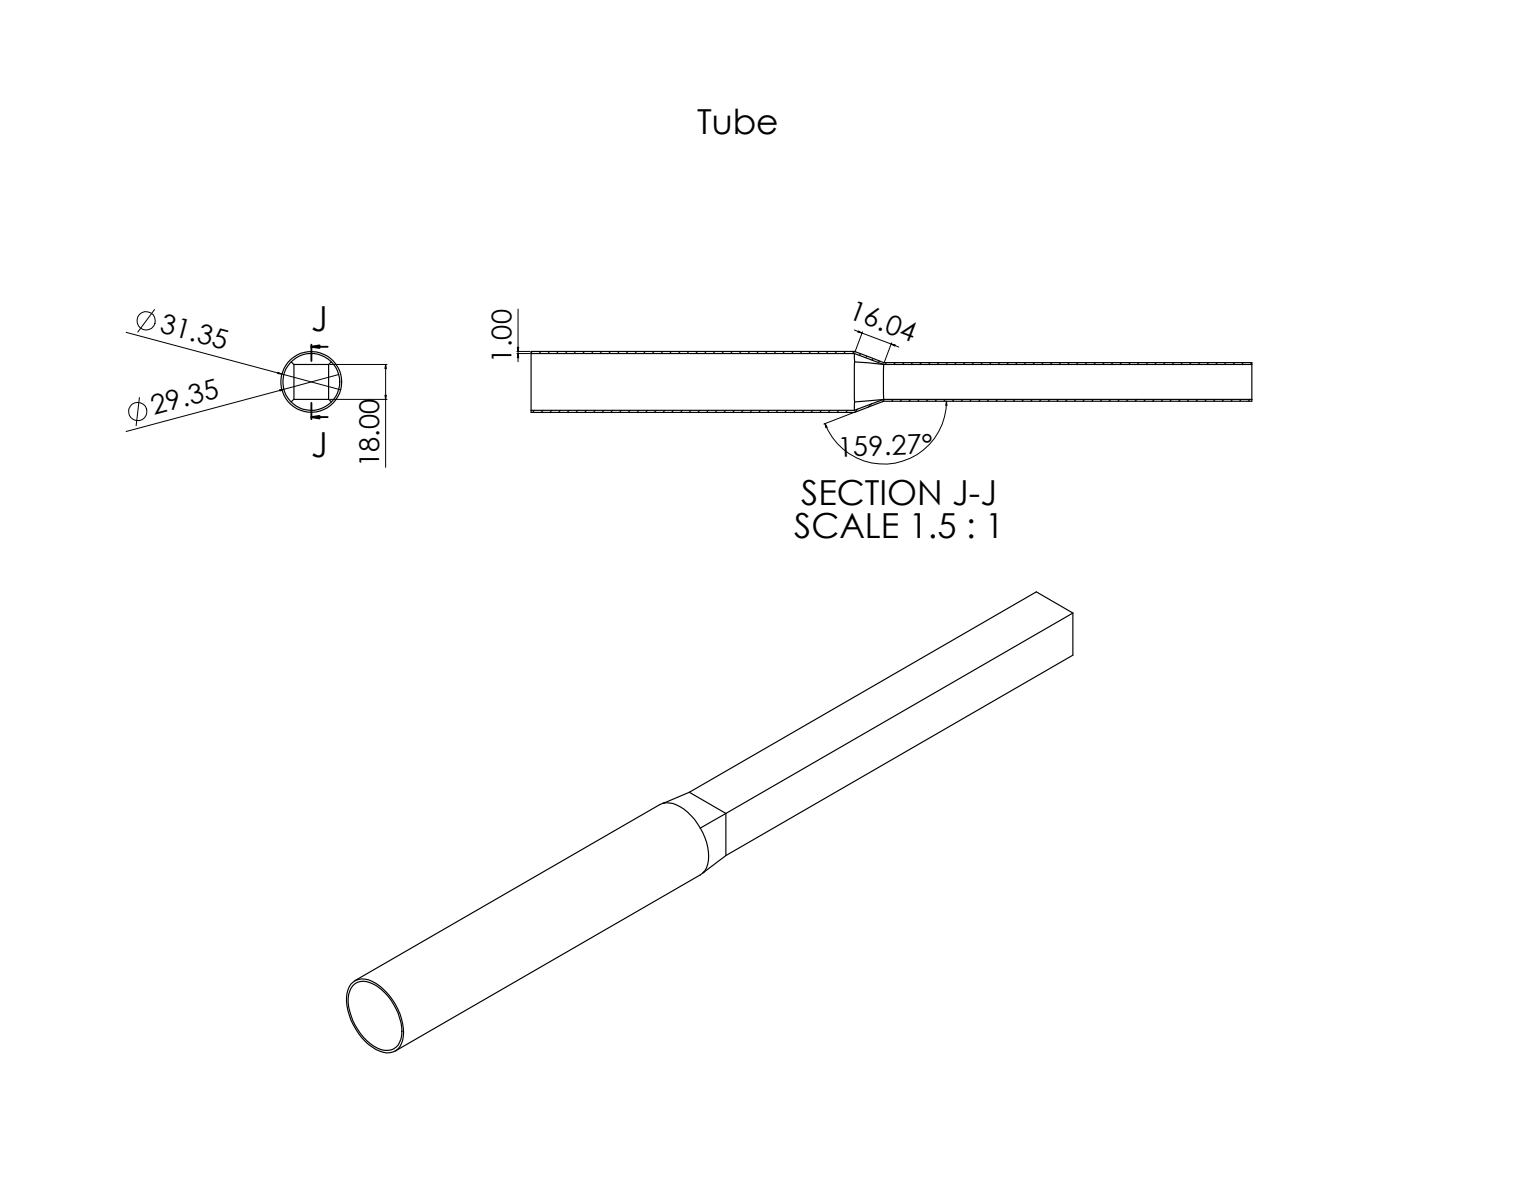
ISO-10303-21;
HEADER;
FILE_DESCRIPTION (('STEP AP214'),
    '1' );
FILE_NAME ('tube.step',
    '2026-10-25T19:19:31',
    ( '' ),
    ( '' ),
    'SwSTEP 2.0',
    'SolidWorks 2025',
    '' );
FILE_SCHEMA (( 'AUTOMOTIVE_DESIGN' ));
ENDSEC;

DATA;
#1=FACE_OUTER_BOUND ( 'NONE', #2199, .T. ) ;
#3=CARTESIAN_POINT ( 'NONE',  ( 6.000509662810415534, -9.000000000000001776, 23.13502399099470708 ) ) ;
#7=CYLINDRICAL_SURFACE ( 'NONE', #5135, 14.67638808697554964 ) ;
#8=ADVANCED_FACE ( 'NONE', ( #6005 ), #1741, .T. ) ;
#10=( NAMED_UNIT ( * ) SI_UNIT ( $, .STERADIAN. ) SOLID_ANGLE_UNIT ( ) );
#14=CARTESIAN_POINT ( 'NONE',  ( 4.154428044945162490, -8.963431230391421423, 23.04275563843252783 ) ) ;
#18=PLANE ( 'NONE',  #4619 ) ;
#25=CARTESIAN_POINT ( 'NONE',  ( 4.399209358691966720, 10.59950146047779995, 28.13666863833444154 ) ) ;
#26=CARTESIAN_POINT ( 'NONE',  ( -0.8333333333332849646, 10.00000000000000000, 23.00000000000000355 ) ) ;
#31=CARTESIAN_POINT ( 'NONE',  ( -9.557272410707511767, 9.557272410707513544, 28.03893107092313031 ) ) ;
#38=CARTESIAN_POINT ( 'NONE',  ( 10.37777353962609972, -10.37777353962564852, 38.05103295300747845 ) ) ;
#39=CARTESIAN_POINT ( 'NONE',  ( 5.954763795926170999, -9.638809746143389035, 25.54536317066256856 ) ) ;
#47=CARTESIAN_POINT ( 'NONE',  ( 9.858401829237470437, -10.19494410001831142, 33.01259202755186095 ) ) ;
#49=ORIENTED_EDGE ( 'NONE', *, *, #1979, .T. ) ;
#50=CARTESIAN_POINT ( 'NONE',  ( 1.902388932222473850, 12.74242197681752486, 33.26151580524048512 ) ) ;
#51=CARTESIAN_POINT ( 'NONE',  ( 11.08488032081242380, 11.08488032081242025, 38.00000000000000000 ) ) ;
#56=ADVANCED_FACE ( 'NONE', ( #3401 ), #273, .T. ) ;
#57=CARTESIAN_POINT ( 'NONE',  ( -10.12138240269938905, -10.27356722921338950, 35.55812462721154787 ) ) ;
#59=STYLED_ITEM('',(#6177),#4119);
#64=CARTESIAN_POINT ( 'NONE',  ( -3.819063922341606521, -14.20304409106748977, 38.16887386538299154 ) ) ;
#66=ORIENTED_EDGE ( 'NONE', *, *, #1371, .T. ) ;
#73=AXIS2_PLACEMENT_3D ( 'NONE', #3304, #3763, #5645 ) ;
#74=CARTESIAN_POINT ( 'NONE',  ( 3.019346778933465369, -14.42236408824967420, 38.33740271606986738 ) ) ;
#87=CARTESIAN_POINT ( 'NONE',  ( -1.016991241531515433, 14.74111653287705792, 38.35393095385146012 ) ) ;
#102=CARTESIAN_POINT ( 'NONE',  ( 0.000000000000000000, 0.000000000000000000, 205.0000000000000568 ) ) ;
#109=CARTESIAN_POINT ( 'NONE',  ( 6.925838250501021420, -10.16165675636470489, 28.06531976343184454 ) ) ;
#115=CARTESIAN_POINT ( 'NONE',  ( -10.37777353962477278, -10.37777353962696303, 38.05103295300743582 ) ) ;
#116=CARTESIAN_POINT ( 'NONE',  ( 10.38144361273100280, -10.38144361273100813, 38.10175261887127363 ) ) ;
#118=PRODUCT_DEFINITION ( 'UNKNOWN', '', #4533, #1451 ) ;
#119=ORIENTED_EDGE ( 'NONE', *, *, #3607, .F. ) ;
#120=CARTESIAN_POINT ( 'NONE',  ( 4.273055220303958457, 9.778265677387498300, 25.59105958838677353 ) ) ;
#121=CARTESIAN_POINT ( 'NONE',  ( 11.73806315776973719, 10.43169748385510687, 38.00000000000000000 ) ) ;
#122=CARTESIAN_POINT ( 'NONE',  ( -13.19705249345109088, -6.492124056757525352, 38.13875458540262997 ) ) ;
#125=CARTESIAN_POINT ( 'NONE',  ( -11.58282027941458381, -3.645499761006322892, 30.69674202529823503 ) ) ;
#129=CARTESIAN_POINT ( 'NONE',  ( 8.309552794738946702, -9.958856949317492990, 22.73823205004162773 ) ) ;
#131=CARTESIAN_POINT ( 'NONE',  ( 0.9493919581231019533, -14.67711297304296281, 38.18288466297301653 ) ) ;
#133=CARTESIAN_POINT ( 'NONE',  ( 6.000548030722291593, 8.999999999999994671, 23.13502304888907446 ) ) ;
#137=CARTESIAN_POINT ( 'NONE',  ( 8.328520801854331523, -12.11088206474084572, 38.20782360758020246 ) ) ;
#146=CARTESIAN_POINT ( 'NONE',  ( 0.8581648076837656847, 9.928243323025451872, 25.63579099555280649 ) ) ;
#147=CARTESIAN_POINT ( 'NONE',  ( 2.164213882025735280, 15.56315586465742484, 38.00000000000000711 ) ) ;
#151=CARTESIAN_POINT ( 'NONE',  ( -13.51119013911330491, -2.923529524533183821, 35.79437308157103814 ) ) ;
#153=CARTESIAN_POINT ( 'NONE',  ( -2.164213882025736613, -15.56315586465742484, 38.00000000000000711 ) ) ;
#156=CARTESIAN_POINT ( 'NONE',  ( 8.964680801521355491, 2.491918585145397991, 23.07363600708416129 ) ) ;
#168=CARTESIAN_POINT ( 'NONE',  ( 1.016991241531512769, -14.74111653287705792, 38.35393095385146012 ) ) ;
#172=FACE_OUTER_BOUND ( 'NONE', #5895, .T. ) ;
#176=B_SPLINE_CURVE_WITH_KNOTS ( 'NONE', 3,
 ( #5640, #360, #5088, #1772, #3271, #6050 ),
 .UNSPECIFIED., .F., .F.,
 ( 4, 2, 4 ),
 ( 2.991083261079382436E-05, 0.007589224902417026838, 0.01514853897222325982 ),
 .UNSPECIFIED. ) ;
#180=CARTESIAN_POINT ( 'NONE',  ( 8.999999999999998224, -9.999999999999998224, 23.00000000000000000 ) ) ;
#181=EDGE_CURVE ( 'NONE', #882, #2297, #5215, .T. ) ;
#186=CARTESIAN_POINT ( 'NONE',  ( 5.819377809724670669, 8.963566137365393871, 22.99383900881164067 ) ) ;
#192=CARTESIAN_POINT ( 'NONE',  ( -9.928243323025453648, 3.951802415609825688E-14, 25.63579099555280294 ) ) ;
#194=CARTESIAN_POINT ( 'NONE',  ( -3.317157231508649495, -9.910574073276151807, 22.73823205004162773 ) ) ;
#195=VECTOR ( 'NONE', #4584, 1000.000000000000000 ) ;
#196=CARTESIAN_POINT ( 'NONE',  ( 13.51119013911330669, 2.923529524533184265, 35.79437308157104525 ) ) ;
#198=LINE ( 'NONE', #2374, #5423 ) ;
#203=CARTESIAN_POINT ( 'NONE',  ( 0.8880320553140116369, -10.89081796499577237, 28.17941898721254645 ) ) ;
#205=DIRECTION ( 'NONE',  ( -0.000000000000000000, -0.000000000000000000, -1.000000000000000000 ) ) ;
#207=CARTESIAN_POINT ( 'NONE',  ( 14.30354638250598498, 3.321916882804190951, 38.17191617598167852 ) ) ;
#219=CARTESIAN_POINT ( 'NONE',  ( 9.999999999999998224, -9.999999999999998224, 23.00000000000000000 ) ) ;
#223=CARTESIAN_POINT ( 'NONE',  ( -9.833810162157899271, -3.423816715609353079, 25.60794618818621160 ) ) ;
#224=EDGE_LOOP ( 'NONE', ( #2924, #3585, #2921, #1569, #6030 ) ) ;
#225=CARTESIAN_POINT ( 'NONE',  ( -8.999999999999998224, 8.999999999999998224, 23.00000000000000000 ) ) ;
#226=CARTESIAN_POINT ( 'NONE',  ( 10.78034266696900012, 2.654236408786700085, 28.16346921039841789 ) ) ;
#231=CARTESIAN_POINT ( 'NONE',  ( -4.003063095775588387, -14.21238549857230993, 38.32638145091770809 ) ) ;
#240=ORIENTED_EDGE ( 'NONE', *, *, #5458, .F. ) ;
#243=CARTESIAN_POINT ( 'NONE',  ( 9.322893336083165394, 9.590870124851308631, 27.95908392747358562 ) ) ;
#244=CARTESIAN_POINT ( 'NONE',  ( 9.916251082295017838, -4.147343260682193389, 22.73823205004162418 ) ) ;
#248=EDGE_CURVE ( 'NONE', #5395, #3300, #425, .T. ) ;
#250=CARTESIAN_POINT ( 'NONE',  ( -10.32656711695238094, -6.095798759547100154, 28.09297316833070113 ) ) ;
#251=VERTEX_POINT ( 'NONE', #3860 ) ;
#254=CARTESIAN_POINT ( 'NONE',  ( 10.46302782743270754, 5.247549479766026259, 28.11481907968152427 ) ) ;
#259=CARTESIAN_POINT ( 'NONE',  ( -5.685785403169735019, -12.74411457810409232, 35.74643938915854591 ) ) ;
#260=ORIENTED_EDGE ( 'NONE', *, *, #822, .T. ) ;
#272=CARTESIAN_POINT ( 'NONE',  ( 7.487361748921665061, 8.967351122863068014, 22.92808036848186504 ) ) ;
#273=B_SPLINE_SURFACE_WITH_KNOTS ( 'NONE', 3, 1, ( 
 ( #5313, #2482, #4370 ),
 ( #121, #3896, #1533 ),
 ( #3311, #5219, #957 ),
 ( #690, #3990, #1683 ),
 ( #2657, #4973, #3555 ),
 ( #774, #4553, #3001 ),
 ( #2602, #5904, #5405 ),
 ( #2062, #1619, #5435 ),
 ( #5474, #4431, #5936 ),
 ( #310, #2189, #4491 ),
 ( #5848, #4517, #1567 ),
 ( #745, #1230, #2626 ),
 ( #4940, #1174, #244 ),
 ( #2573, #1596, #3519 ),
 ( #3468, #3492, #5381 ),
 ( #1204, #1145, #5001 ),
 ( #4464, #1120, #3063 ),
 ( #2116, #219, #4911 ) ),
 .UNSPECIFIED., .F., .F., .F.,
 ( 4, 2, 2, 2, 2, 2, 2, 2, 4 ),
 ( 2, 1, 2 ),
 ( 0.000000000000000000, 0.1250000000000000000, 0.2500000000000000000, 0.3750000000000000000, 0.4999999999999999445, 0.6250000000000000000, 0.7500000000000000000, 0.8750000000000000000, 1.000000000000000000 ),
 ( 0.000000000000000000, 1.000000000000000000, 1.017451196663891722 ),
 .UNSPECIFIED. ) ;
#281=CARTESIAN_POINT ( 'NONE',  ( -9.793760812180220654, 8.539139919159236314, 27.99841606626185353 ) ) ;
#293=VECTOR ( 'NONE', #3601, 1000.000000000000000 ) ;
#294=CARTESIAN_POINT ( 'NONE',  ( 2.830884587392746621, -12.60026679007841466, 33.25110354061416018 ) ) ;
#297=VECTOR ( 'NONE', #4183, 1000.000000000000000 ) ;
#298=ORIENTED_EDGE ( 'NONE', *, *, #2594, .T. ) ;
#303=CARTESIAN_POINT ( 'NONE',  ( 15.67638808697555142, 1.919803849290630886E-15, 205.0000000000000568 ) ) ;
#304=CARTESIAN_POINT ( 'NONE',  ( -9.999999999999998224, 1.666666666666715368, 23.00000000000000000 ) ) ;
#306=ORIENTED_EDGE ( 'NONE', *, *, #668, .F. ) ;
#310=CARTESIAN_POINT ( 'NONE',  ( 15.67638808697555142, -1.082228759108216254, 38.00000000000000711 ) ) ;
#314=CARTESIAN_POINT ( 'NONE',  ( 8.964120815521452457, -3.322922547535530846, 23.06129036953744915 ) ) ;
#315=CARTESIAN_POINT ( 'NONE',  ( -10.78034266696900190, 2.654236408786762702, 28.16346921039841078 ) ) ;
#317=CARTESIAN_POINT ( 'NONE',  ( -10.08321815271042432, 9.378998278013591872, 27.91486726096250948 ) ) ;
#323=EDGE_LOOP ( 'NONE', ( #4367, #5379, #3695, #5284 ) ) ;
#325=CARTESIAN_POINT ( 'NONE',  ( -6.737147714782520502, -13.11522978513662530, 38.26633100282688105 ) ) ;
#330=PLANE ( 'NONE',  #3954 ) ;
#333=CARTESIAN_POINT ( 'NONE',  ( -13.97471987708211216, -7.178663235509280760, 37.99999999999999289 ) ) ;
#336=EDGE_LOOP ( 'NONE', ( #5694, #5269, #1258, #942 ) ) ;
#340=( NAMED_UNIT ( * ) PLANE_ANGLE_UNIT ( ) SI_UNIT ( $, .RADIAN. ) );
#341=CARTESIAN_POINT ( 'NONE',  ( 8.965240787521256749, -1.660914622755447212, 23.08598164463087343 ) ) ;
#342=CARTESIAN_POINT ( 'NONE',  ( -11.98089146579573061, 5.533593864557679431, 33.20390238845318720 ) ) ;
#344=CARTESIAN_POINT ( 'NONE',  ( -8.662324224478984647, 10.23352841777492017, 30.54531597708798074 ) ) ;
#351=CARTESIAN_POINT ( 'NONE',  ( -8.539139919159234537, -9.793760812180220654, 27.99841606626185353 ) ) ;
#353=CARTESIAN_POINT ( 'NONE',  ( 10.37777353962609972, -10.37777353962564852, 38.05103295300747845 ) ) ;
#359=CARTESIAN_POINT ( 'NONE',  ( -9.916251082295017838, 4.147343260682193389, 22.73823205004162418 ) ) ;
#360=CARTESIAN_POINT ( 'NONE',  ( 10.19629538392542933, -10.19629538388540446, 35.54424335298407556 ) ) ;
#363=PLANE ( 'NONE',  #2855 ) ;
#365=CARTESIAN_POINT ( 'NONE',  ( 2.411881101062863575, 14.48475173028204566, 38.17746263717076971 ) ) ;
#369=CARTESIAN_POINT ( 'NONE',  ( 12.81596724893641515, -0.9505942623812210224, 33.26667497053200151 ) ) ;
#370=CARTESIAN_POINT ( 'NONE',  ( -8.963566137365393871, 5.819377809724669781, 22.99383900881164067 ) ) ;
#374=CARTESIAN_POINT ( 'NONE',  ( -2.035738251814317223, 14.63232105816060979, 38.34842656511671066 ) ) ;
#380=CARTESIAN_POINT ( 'NONE',  ( -9.419333092093008730, -9.933255351449998827, 30.50691708577706152 ) ) ;
#384=ORIENTED_EDGE ( 'NONE', *, *, #2250, .F. ) ;
#388=CARTESIAN_POINT ( 'NONE',  ( -9.999999999999998224, 6.666666666666692720, 23.00000000000000000 ) ) ;
#399=CARTESIAN_POINT ( 'NONE',  ( 14.63234267792704557, -2.035630462091353898, 38.34842398122204798 ) ) ;
#402=CARTESIAN_POINT ( 'NONE',  ( -9.908812303639313868, 1.716658579843643118, 25.63028407385522911 ) ) ;
#405=CARTESIAN_POINT ( 'NONE',  ( -8.321944142006520551, 8.970286642449650572, 22.89273687632151066 ) ) ;
#412=CARTESIAN_POINT ( 'NONE',  ( -8.926511697459380557, -11.12726264164139600, 35.63515070857870626 ) ) ;
#420=CARTESIAN_POINT ( 'NONE',  ( -13.47611570251764590, -8.069545871843427420, 37.99999999999998579 ) ) ;
#423=CARTESIAN_POINT ( 'NONE',  ( -9.999999999999998224, -9.999999999999998224, 23.00000000000000000 ) ) ;
#425=LINE ( 'NONE', #3727, #495 ) ;
#427=CARTESIAN_POINT ( 'NONE',  ( 11.85339260696609109, 0.9193131588475963456, 30.72304697887226510 ) ) ;
#430=CARTESIAN_POINT ( 'NONE',  ( -5.685785403169716368, 12.74411457810409587, 35.74643938915853880 ) ) ;
#436=CARTESIAN_POINT ( 'NONE',  ( -10.63625351335941538, -9.632247231687289357, 35.59852902770368388 ) ) ;
#437=CARTESIAN_POINT ( 'NONE',  ( -14.67638808697506114, 0.4806947631990008407, 38.18288438803430296 ) ) ;
#450=ORIENTED_EDGE ( 'NONE', *, *, #856, .T. ) ;
#452=FACE_OUTER_BOUND ( 'NONE', #336, .T. ) ;
#453=CARTESIAN_POINT ( 'NONE',  ( -0.9493919581226956117, 14.67711297304298768, 38.18288466297298811 ) ) ;
#458=CARTESIAN_POINT ( 'NONE',  ( -3.423816715609354411, 9.833810162157899271, 25.60794618818621160 ) ) ;
#464=VERTEX_POINT ( 'NONE', #2022 ) ;
#467=CARTESIAN_POINT ( 'NONE',  ( -8.983694681928700021, -9.994658916190591214, 22.80938439471025703 ) ) ;
#486=CARTESIAN_POINT ( 'NONE',  ( 5.533593864557655451, -11.98089146579573061, 33.20390238845318720 ) ) ;
#487=APPLICATION_CONTEXT ( 'automotive_design' ) ;
#488=EDGE_LOOP ( 'NONE', ( #3553, #1325 ) ) ;
#490=FACE_OUTER_BOUND ( 'NONE', #2075, .T. ) ;
#495=VECTOR ( 'NONE', #5181, 1000.000000000000000 ) ;
#497=CARTESIAN_POINT ( 'NONE',  ( 9.590870124851305079, -9.322893336083168947, 27.95908392747358562 ) ) ;
#498=VECTOR ( 'NONE', #1818, 1000.000000000000000 ) ;
#500=CARTESIAN_POINT ( 'NONE',  ( 4.003063095775587499, 14.21238549857231170, 38.32638145091770809 ) ) ;
#502=CARTESIAN_POINT ( 'NONE',  ( 0.8333333333333816650, 9.999999999999998224, 23.00000000000000000 ) ) ;
#514=CARTESIAN_POINT ( 'NONE',  ( 10.99573437649350538, 9.772747244158498603, 38.14042781937034476 ) ) ;
#515=CARTESIAN_POINT ( 'NONE',  ( 4.709709529607406964, -13.90855959397108954, 38.16103891068024012 ) ) ;
#523=CARTESIAN_POINT ( 'NONE',  ( 9.245260337044127752, -9.269614772507658529, 25.40693856330804934 ) ) ;
#526=CARTESIAN_POINT ( 'NONE',  ( -9.999999999999998224, -9.999999999999998224, 23.00000000000000000 ) ) ;
#532=CARTESIAN_POINT ( 'NONE',  ( 9.933255351449995274, -9.419333092093014059, 30.50691708577705796 ) ) ;
#534=CARTESIAN_POINT ( 'NONE',  ( 6.095889600840177280, 10.32655419438761690, 28.09296952102860701 ) ) ;
#535=CARTESIAN_POINT ( 'NONE',  ( 6.642184745761470666, 9.939337621248920840, 22.73823205004162418 ) ) ;
#539=CARTESIAN_POINT ( 'NONE',  ( -10.38144361273100635, -10.38144361273100458, 38.10175261887127363 ) ) ;
#541=DIRECTION ( 'NONE',  ( -0.000000000000000000, -0.000000000000000000, -1.000000000000000000 ) ) ;
#542=CARTESIAN_POINT ( 'NONE',  ( 9.676903716103607778, -11.04476983075560348, 38.07288907902118069 ) ) ;
#547=CARTESIAN_POINT ( 'NONE',  ( 12.71058384521441198, -7.353037798771444145, 38.12486502407008970 ) ) ;
#548=CARTESIAN_POINT ( 'NONE',  ( 4.954970571217797826, -13.90079966151758306, 38.30990426830500439 ) ) ;
#562=CARTESIAN_POINT ( 'NONE',  ( -0.9833031778629136577, 13.77854189090673742, 35.81030296219172726 ) ) ;
#569=CARTESIAN_POINT ( 'NONE',  ( -11.71459457793454995, -6.400384853991337941, 33.18278774224378225 ) ) ;
#572=CARTESIAN_POINT ( 'NONE',  ( -9.166666666666673180, -9.999999999999998224, 23.00000000000000000 ) ) ;
#576=DIRECTION ( 'NONE',  ( -0.000000000000000000, -0.000000000000000000, -1.000000000000000000 ) ) ;
#586=CARTESIAN_POINT ( 'NONE',  ( 7.077301327650767249, -10.77711034800893231, 30.61076202992614625 ) ) ;
#587=VECTOR ( 'NONE', #3050, 1000.000000000000000 ) ;
#595=CARTESIAN_POINT ( 'NONE',  ( 10.50531938289192624, -7.869812776064898152, 30.57803900350706527 ) ) ;
#599=CARTESIAN_POINT ( 'NONE',  ( 3.531766105781286580, 10.70751178813581461, 28.15279191876807374 ) ) ;
#605=EDGE_CURVE ( 'NONE', #2868, #2500, #2363, .T. ) ;
#606=CARTESIAN_POINT ( 'NONE',  ( -10.59948853791303414, -4.399300199984967463, 28.13666499103235452 ) ) ;
#610=CARTESIAN_POINT ( 'NONE',  ( -8.333333333333348136, -9.999999999999998224, 23.00000000000000000 ) ) ;
#613=CARTESIAN_POINT ( 'NONE',  ( 10.12138240269938905, 10.27356722921338950, 35.55812462721154787 ) ) ;
#615=CIRCLE ( 'NONE', #5164, 15.67638808697555142 ) ;
#619=CARTESIAN_POINT ( 'NONE',  ( 8.999999999999994671, -3.000437278975552235, 23.18288419282212587 ) ) ;
#621=CARTESIAN_POINT ( 'NONE',  ( 5.247549479766027147, -10.46302782743270754, 28.11481907968152427 ) ) ;
#624=ORIENTED_EDGE ( 'NONE', *, *, #3473, .T. ) ;
#628=CARTESIAN_POINT ( 'NONE',  ( -10.19629538388490353, -10.19629538392591428, 35.54424335298404714 ) ) ;
#632=CARTESIAN_POINT ( 'NONE',  ( 0.8880320553140821360, 10.89081796499577059, 28.17941898721253580 ) ) ;
#633=CARTESIAN_POINT ( 'NONE',  ( 7.178663235509286977, 13.97471987708211394, 38.00000000000000000 ) ) ;
#638=CARTESIAN_POINT ( 'NONE',  ( -13.68733454931619953, 1.968046268140568156, 35.80501179064255268 ) ) ;
#640=CARTESIAN_POINT ( 'NONE',  ( 3.317157231508561122, -9.910574073276151807, 22.73823205004162773 ) ) ;
#642=CARTESIAN_POINT ( 'NONE',  ( 12.45812449473958949, 3.759289558891020455, 33.24069098933200905 ) ) ;
#646=EDGE_CURVE ( 'NONE', #1950, #464, #2666, .T. ) ;
#647=CARTESIAN_POINT ( 'NONE',  ( 2.742560498089724241, -11.69030472852370828, 30.70728637550628903 ) ) ;
#654=CARTESIAN_POINT ( 'NONE',  ( 0.000000000000000000, 0.000000000000000000, 38.00000000000000000 ) ) ;
#657=ORIENTED_EDGE ( 'NONE', *, *, #2551, .F. ) ;
#663=CARTESIAN_POINT ( 'NONE',  ( -12.60026679007840933, -2.830884587392748397, 33.25110354061415308 ) ) ;
#664=ORIENTED_EDGE ( 'NONE', *, *, #2969, .F. ) ;
#665=CARTESIAN_POINT ( 'NONE',  ( 1.082228759108211813, -15.67638808697554786, 38.00000000000000711 ) ) ;
#668=EDGE_CURVE ( 'NONE', #5813, #4909, #2649, .T. ) ;
#669=CARTESIAN_POINT ( 'NONE',  ( 12.74240908541723805, 1.902479615894477449, 33.26151609189631841 ) ) ;
#671=CARTESIAN_POINT ( 'NONE',  ( 8.999999999988068211, 9.000000000000005329, 23.06137295785747554 ) ) ;
#675=EDGE_CURVE ( 'NONE', #4909, #1654, #1700, .T. ) ;
#676=CARTESIAN_POINT ( 'NONE',  ( -4.273055220303960233, -9.778265677387510735, 25.59105958838677708 ) ) ;
#684=( GEOMETRIC_REPRESENTATION_CONTEXT ( 3 ) GLOBAL_UNCERTAINTY_ASSIGNED_CONTEXT ( ( #3684 ) ) GLOBAL_UNIT_ASSIGNED_CONTEXT ( ( #1802, #340, #1744 ) ) REPRESENTATION_CONTEXT ( 'NONE', 'WORKASPACE' ) );
#689=CARTESIAN_POINT ( 'NONE',  ( 8.159736356077655017, 11.57174281757876955, 35.66679457777021156 ) ) ;
#690=CARTESIAN_POINT ( 'NONE',  ( 13.47611570251764768, 8.069545871843432749, 37.99999999999999289 ) ) ;
#692=ORIENTED_EDGE ( 'NONE', *, *, #2352, .F. ) ;
#694=CARTESIAN_POINT ( 'NONE',  ( -12.81596724893641337, 1.499651672263871603E-14, 33.26667497053200151 ) ) ;
#696=ORIENTED_EDGE ( 'NONE', *, *, #3568, .F. ) ;
#702=CARTESIAN_POINT ( 'NONE',  ( 9.708537589994000072, 5.113933401365464704, 25.56820946177495557 ) ) ;
#711=CARTESIAN_POINT ( 'NONE',  ( -1.117102909420315718E-14, -13.77854189090673742, 35.81030296219173437 ) ) ;
#714=CARTESIAN_POINT ( 'NONE',  ( 14.58318388806640442, 1.909955344851026027, 38.18050947768620063 ) ) ;
#716=ADVANCED_FACE ( 'NONE', ( #885 ), #3690, .T. ) ;
#717=CARTESIAN_POINT ( 'NONE',  ( -10.00265588554885454, -10.00265588554885454, 33.03935750738951782 ) ) ;
#721=CARTESIAN_POINT ( 'NONE',  ( 7.610208295502498999, 9.462636878983097688, 25.48187184588751464 ) ) ;
#725=CARTESIAN_POINT ( 'NONE',  ( -8.964120776013636771, -3.322926169935023655, 23.06129021161080317 ) ) ;
#728=CARTESIAN_POINT ( 'NONE',  ( 13.50805179034378689, 5.845970755595363499, 38.28811402100272687 ) ) ;
#733=CARTESIAN_POINT ( 'NONE',  ( -4.807771419025854698, -13.07374771013670411, 35.76776546669864132 ) ) ;
#735=CARTESIAN_POINT ( 'NONE',  ( -8.999999999999994671, 3.000437278975516708, 23.18288419282211521 ) ) ;
#744=CARTESIAN_POINT ( 'NONE',  ( 9.632247231687292910, 10.63625351335941716, 35.59852902770369809 ) ) ;
#745=CARTESIAN_POINT ( 'NONE',  ( 15.12434353048566571, -4.260267006495016773, 38.00000000000000711 ) ) ;
#746=CARTESIAN_POINT ( 'NONE',  ( -15.67638808697555142, -2.609965535188016420E-15, 38.00000000000000711 ) ) ;
#750=CARTESIAN_POINT ( 'NONE',  ( -10.67320828294309898, 8.785766938566926143, 33.09220912812762094 ) ) ;
#752=CARTESIAN_POINT ( 'NONE',  ( -10.27356722921338950, 10.12138240269938905, 35.55812462721154787 ) ) ;
#754=CARTESIAN_POINT ( 'NONE',  ( 10.23352841777492017, 8.662324224478986423, 30.54531597708798074 ) ) ;
#758=B_SPLINE_CURVE_WITH_KNOTS ( 'NONE', 3,
 ( #38, #2893, #943, #4797, #547, #2366, #1364, #5699, #2425, #1916, #4261, #3269, #2864, #4768 ),
 .UNSPECIFIED., .F., .F.,
 ( 4, 2, 2, 2, 2, 2, 4 ),
 ( 2.453269466693398698E-18, 0.002860246893306488992, 0.004290370339959730453, 0.005720493786612971913, 0.008580740679919452232, 0.01001086412657269456, 0.01144098757322593515 ),
 .UNSPECIFIED. ) ;
#760=CARTESIAN_POINT ( 'NONE',  ( -3.759380242563084451, -12.45811160333930800, 33.24069127598783524 ) ) ;
#761=ORIENTED_EDGE ( 'NONE', *, *, #4032, .F. ) ;
#766=VECTOR ( 'NONE', #3692, 1000.000000000000000 ) ;
#768=PRODUCT_CONTEXT ( 'NONE', #487, 'mechanical' ) ;
#770=CARTESIAN_POINT ( 'NONE',  ( -9.969668718019493170, -9.144590365090015993, 22.73823205004162418 ) ) ;
#774=CARTESIAN_POINT ( 'NONE',  ( 14.79903580929011753, 5.273949241992679227, 38.00000000000000711 ) ) ;
#779=ADVANCED_FACE ( 'NONE', ( #5517 ), #330, .T. ) ;
#783=CARTESIAN_POINT ( 'NONE',  ( -10.99573437649350183, 9.772747244158500379, 38.14042781937034476 ) ) ;
#785=CARTESIAN_POINT ( 'NONE',  ( -9.772747244158496827, 10.99573437649350538, 38.14042781937034476 ) ) ;
#795=CARTESIAN_POINT ( 'NONE',  ( -7.228600378928581982, -11.39263409468387422, 33.15620577507543487 ) ) ;
#801=CARTESIAN_POINT ( 'NONE',  ( 0.000000000000000000, 0.000000000000000000, 38.00000000000000000 ) ) ;
#805=CARTESIAN_POINT ( 'NONE',  ( -9.999999999999998224, 3.333333333333377890, 23.00000000000000000 ) ) ;
#814=CARTESIAN_POINT ( 'NONE',  ( 13.77854189090674097, -0.9833031778629309771, 35.81030296219172726 ) ) ;
#815=CARTESIAN_POINT ( 'NONE',  ( -11.03292118881348394, 8.007183658747754507, 33.12420745160153501 ) ) ;
#817=CARTESIAN_POINT ( 'NONE',  ( -6.248091806769195955, 11.02058084744346189, 30.63788045528724524 ) ) ;
#820=CARTESIAN_POINT ( 'NONE',  ( 8.999999999999994671, 6.000509662810391553, 23.13502399099459339 ) ) ;
#822=EDGE_CURVE ( 'NONE', #5813, #2500, #2325, .T. ) ;
#826=CARTESIAN_POINT ( 'NONE',  ( -7.487361748921665061, -8.967351122863068014, 22.92808036848186859 ) ) ;
#834=CARTESIAN_POINT ( 'NONE',  ( -9.999999999999998224, 5.833333333333365012, 23.00000000000000000 ) ) ;
#839=CARTESIAN_POINT ( 'NONE',  ( -6.488003555186317328, 13.19914683770227093, 38.13881399654477633 ) ) ;
#840=CARTESIAN_POINT ( 'NONE',  ( 10.85317354580219629, -1.776706711792237492, 28.17414650202875137 ) ) ;
#841=CARTESIAN_POINT ( 'NONE',  ( -8.963498645742985715, 4.986905650496099796, 23.01829711214647745 ) ) ;
#843=CARTESIAN_POINT ( 'NONE',  ( -5.390571672161838634, 11.22195964661421819, 30.65936073406735574 ) ) ;
#846=CARTESIAN_POINT ( 'NONE',  ( -14.65251043020005461, 0.9663357036150521662, 38.18273246053422554 ) ) ;
#856=EDGE_CURVE ( 'NONE', #1594, #1863, #4862, .T. ) ;
#857=CARTESIAN_POINT ( 'NONE',  ( -15.12434353048566216, -4.260267006495012332, 37.99999999999999289 ) ) ;
#863=CARTESIAN_POINT ( 'NONE',  ( -11.08488032081242558, -11.08488032081241847, 38.00000000000000000 ) ) ;
#864=CARTESIAN_POINT ( 'NONE',  ( 1.937269431830858979, 14.55597330376932774, 38.18000980160653768 ) ) ;
#865=CARTESIAN_POINT ( 'NONE',  ( 13.07374771013670589, -4.807771419025858251, 35.76776546669863421 ) ) ;
#866=VECTOR ( 'NONE', #2323, 1000.000000000000000 ) ;
#867=CARTESIAN_POINT ( 'NONE',  ( -12.24723121994939135, 4.666652649023722788, 33.22501677959694177 ) ) ;
#871=CARTESIAN_POINT ( 'NONE',  ( -7.869812776064877724, 10.50531938289192624, 30.57803900350706172 ) ) ;
#879=CARTESIAN_POINT ( 'NONE',  ( -9.322893336083163618, -9.590870124851308631, 27.95908392747358917 ) ) ;
#882=VERTEX_POINT ( 'NONE', #2422 ) ;
#885=FACE_OUTER_BOUND ( 'NONE', #1773, .T. ) ;
#888=CARTESIAN_POINT ( 'NONE',  ( -12.35760627049922000, -9.696021465980068754, 37.99999999999998579 ) ) ;
#891=VECTOR ( 'NONE', #1166, 1000.000000000000000 ) ;
#895=EDGE_CURVE ( 'NONE', #2972, #5932, #3846, .T. ) ;
#900=CARTESIAN_POINT ( 'NONE',  ( 9.778265677387498300, -4.273055220303958457, 25.59105958838677353 ) ) ;
#901=CIRCLE ( 'NONE', #1670, 15.67638808697555142 ) ;
#903=ADVANCED_FACE ( 'NONE', ( #2395 ), #7, .F. ) ;
#904=CARTESIAN_POINT ( 'NONE',  ( -8.432782529159778662, 9.370308598635419983, 25.44727941985334496 ) ) ;
#908=CARTESIAN_POINT ( 'NONE',  ( -14.55721289103182237, 1.928061058260225558, 38.18004976450266952 ) ) ;
#909=CARTESIAN_POINT ( 'NONE',  ( -9.086997423426605991, -11.58116666691846852, 38.17633527770230017 ) ) ;
#910=EDGE_LOOP ( 'NONE', ( #49, #1213, #66, #5315 ) ) ;
#920=DIRECTION ( 'NONE',  ( -0.000000000000000000, -0.000000000000000000, -1.000000000000000000 ) ) ;
#925=CARTESIAN_POINT ( 'NONE',  ( 11.22195964661421641, -5.390571672161878602, 30.65936073406735218 ) ) ;
#928=CARTESIAN_POINT ( 'NONE',  ( -8.328520801854338629, 12.11088206474084750, 38.20782360758020957 ) ) ;
#929=CARTESIAN_POINT ( 'NONE',  ( -11.08488032081242025, 11.08488032081242203, 38.00000000000000000 ) ) ;
#936=VERTEX_POINT ( 'NONE', #3385 ) ;
#942=ORIENTED_EDGE ( 'NONE', *, *, #895, .F. ) ;
#943=CARTESIAN_POINT ( 'NONE',  ( 11.66987820548568600, -8.950926204225938321, 38.09167945787535103 ) ) ;
#944=CARTESIAN_POINT ( 'NONE',  ( 8.432782529159780438, -9.370308598635425312, 25.44727941985334851 ) ) ;
#955=ORIENTED_EDGE ( 'NONE', *, *, #646, .F. ) ;
#956=CARTESIAN_POINT ( 'NONE',  ( 8.830123324796599503E-15, 13.77854189090673742, 35.81030296219172726 ) ) ;
#957=CARTESIAN_POINT ( 'NONE',  ( 9.958856949317492990, 8.309552794738946702, 22.73823205004162418 ) ) ;
#966=CARTESIAN_POINT ( 'NONE',  ( -10.23352841777491840, -8.662324224478982870, 30.54531597708798074 ) ) ;
#973=CARTESIAN_POINT ( 'NONE',  ( 5.161660887237665918, -13.74708875321000789, 38.15586426248330554 ) ) ;
#978=DIRECTION ( 'NONE',  ( 1.000000000000000000, 0.000000000000000000, 0.000000000000000000 ) ) ;
#983=CARTESIAN_POINT ( 'NONE',  ( 3.759289558891017347, -12.45812449473959127, 33.24069098933200195 ) ) ;
#984=ORIENTED_EDGE ( 'NONE', *, *, #4331, .T. ) ;
#994=CARTESIAN_POINT ( 'NONE',  ( 4.666652649023724564, 12.24723121994938779, 33.22501677959694177 ) ) ;
#996=CARTESIAN_POINT ( 'NONE',  ( -3.317157231508560677, 9.910574073276151807, 22.73823205004162418 ) ) ;
#1001=AXIS2_PLACEMENT_3D ( 'NONE', #5430, #3956, #3984 ) ;
#1002=CARTESIAN_POINT ( 'NONE',  ( -9.618700053625529378, -10.13908112636437053, 30.46372964425718521 ) ) ;
#1003=CARTESIAN_POINT ( 'NONE',  ( -6.666666666666693608, -9.999999999999998224, 23.00000000000000000 ) ) ;
#1008=CARTESIAN_POINT ( 'NONE',  ( -7.765009959109524296, -12.46305503907367829, 38.11687012676383546 ) ) ;
#1014=FACE_BOUND ( 'NONE', #3004, .T. ) ;
#1016=CARTESIAN_POINT ( 'NONE',  ( 7.393143600131246274, -12.01612071878465571, 35.69844150329611665 ) ) ;
#1020=DIRECTION ( 'NONE',  ( 0.000000000000000000, 1.000000000000000000, 0.000000000000000000 ) ) ;
#1025=DIRECTION ( 'NONE',  ( 0.000000000000000000, -1.000000000000000000, 0.000000000000000000 ) ) ;
#1026=ORIENTED_EDGE ( 'NONE', *, *, #4032, .T. ) ;
#1027=CARTESIAN_POINT ( 'NONE',  ( 3.080172029080881894E-14, 10.89081796499577237, 28.17941898721253580 ) ) ;
#1028=CARTESIAN_POINT ( 'NONE',  ( -1.657983872361815658, 9.902916272933978803, 22.73823205004162418 ) ) ;
#1032=CARTESIAN_POINT ( 'NONE',  ( -12.01612071878465393, -7.393143600131249826, 35.69844150329610954 ) ) ;
#1033=CARTESIAN_POINT ( 'NONE',  ( -5.809855716632679190, -9.930636381741159369, 22.73823205004162773 ) ) ;
#1034=CARTESIAN_POINT ( 'NONE',  ( -9.306281718482047438, 9.306281718482050991, 25.54332486258997292 ) ) ;
#1035=CARTESIAN_POINT ( 'NONE',  ( -4.735139425639592226, -13.92517021172167624, 38.16137691020122702 ) ) ;
#1037=CARTESIAN_POINT ( 'NONE',  ( -9.999999999999998224, -9.999999999999998224, -167.0000000000000284 ) ) ;
#1040=ADVANCED_FACE ( 'NONE', ( #2741 ), #363, .F. ) ;
#1044=CARTESIAN_POINT ( 'NONE',  ( 5.845970755595360835, -13.50805179034379400, 38.28811402100272687 ) ) ;
#1051=EDGE_CURVE ( 'NONE', #1654, #5395, #2655, .T. ) ;
#1053=CARTESIAN_POINT ( 'NONE',  ( 9.977717576970368540, -7.732441893382042686, 28.03187055541259909 ) ) ;
#1055=ORIENTED_EDGE ( 'NONE', *, *, #1408, .F. ) ;
#1056=CARTESIAN_POINT ( 'NONE',  ( 1.968046268140572819, 13.68733454931619775, 35.80501179064255268 ) ) ;
#1057=CARTESIAN_POINT ( 'NONE',  ( -1.082228759108214478, 15.67638808697554786, 38.00000000000000711 ) ) ;
#1063=CARTESIAN_POINT ( 'NONE',  ( -13.77854189090673742, -0.9833031778629152120, 35.81030296219172726 ) ) ;
#1067=CARTESIAN_POINT ( 'NONE',  ( 9.166666666666657193, -9.999999999999998224, 23.00000000000000000 ) ) ;
#1070=CARTESIAN_POINT ( 'NONE',  ( 8.999999999999998224, 8.999999999999998224, 23.00000000000000000 ) ) ;
#1071=DIRECTION ( 'NONE',  ( 0.000000000000000000, 0.000000000000000000, -1.000000000000000000 ) ) ;
#1079=CARTESIAN_POINT ( 'NONE',  ( 5.819383256046889663, -8.963566061094551785, 22.99383858586043772 ) ) ;
#1084=CARTESIAN_POINT ( 'NONE',  ( 10.54244016040620835, -10.54244016040621190, 30.50000000000000000 ) ) ;
#1087=PLANE ( 'NONE',  #2380 ) ;
#1092=CARTESIAN_POINT ( 'NONE',  ( 5.113933401365548193, 9.708537589994000072, 25.56820946177495557 ) ) ;
#1099=CARTESIAN_POINT ( 'NONE',  ( -13.33506331686137614, -3.878911688431557536, 35.78373290693654951 ) ) ;
#1103=CARTESIAN_POINT ( 'NONE',  ( 9.696021465980065202, -12.35760627049922356, 37.99999999999999289 ) ) ;
#1105=CARTESIAN_POINT ( 'NONE',  ( 14.42236408824967242, 3.019346778933472031, 38.33740271606986738 ) ) ;
#1108=ORIENTED_EDGE ( 'NONE', *, *, #3013, .T. ) ;
#1111=CARTESIAN_POINT ( 'NONE',  ( 1.716690548177164821, -9.908812100099977371, 25.63028262842344773 ) ) ;
#1114=CARTESIAN_POINT ( 'NONE',  ( 10.72018218391672661, 10.03536489533503762, 38.06196296973745774 ) ) ;
#1116=CARTESIAN_POINT ( 'NONE',  ( 9.999999999999998224, 9.999999999999998224, -167.0000000000000284 ) ) ;
#1119=CARTESIAN_POINT ( 'NONE',  ( 6.925743867604852610, 10.16167434176051643, 28.06532504456334109 ) ) ;
#1120=CARTESIAN_POINT ( 'NONE',  ( 9.999999999999998224, -9.166666666666673180, 23.00000000000000000 ) ) ;
#1126=CARTESIAN_POINT ( 'NONE',  ( -9.708537589994000072, -5.113933401365464704, 25.56820946177495912 ) ) ;
#1127=ORIENTED_EDGE ( 'NONE', *, *, #3568, .T. ) ;
#1128=CARTESIAN_POINT ( 'NONE',  ( -9.696021465980074083, -12.35760627049922178, 38.00000000000000000 ) ) ;
#1130=CARTESIAN_POINT ( 'NONE',  ( 13.90079966151757951, 4.954970571217797826, 38.30990426830500439 ) ) ;
#1134=CARTESIAN_POINT ( 'NONE',  ( -2.763109891354090380E-14, -11.85339260696609465, 30.72304697887227221 ) ) ;
#1136=DIRECTION ( 'NONE',  ( 0.000000000000000000, 0.000000000000000000, -1.000000000000000000 ) ) ;
#1138=CARTESIAN_POINT ( 'NONE',  ( -8.999999999999998224, 8.999999999999998224, -167.0000000000000284 ) ) ;
#1144=CARTESIAN_POINT ( 'NONE',  ( 10.13908112636436343, 9.618700053625531154, 30.46372964425718521 ) ) ;
#1145=CARTESIAN_POINT ( 'NONE',  ( 9.999999999999998224, -8.333333333333348136, 23.00000000000000000 ) ) ;
#1147=CARTESIAN_POINT ( 'NONE',  ( -11.42333844578496915, -4.533051537554476873, 30.68084101284746623 ) ) ;
#1148=ORIENTED_EDGE ( 'NONE', *, *, #605, .F. ) ;
#1154=CARTESIAN_POINT ( 'NONE',  ( 10.67327843797381171, 8.785602912694963962, 33.09221060678261495 ) ) ;
#1157=VERTEX_POINT ( 'NONE', #3209 ) ;
#1159=DIRECTION ( 'NONE',  ( 1.000000000000000000, 0.000000000000000000, 0.000000000000000000 ) ) ;
#1160=CARTESIAN_POINT ( 'NONE',  ( -4.721144251037624463E-14, -8.965668681055127820, 23.09216300389307364 ) ) ;
#1162=EDGE_CURVE ( 'NONE', #3749, #1654, #5740, .T. ) ;
#1166=DIRECTION ( 'NONE',  ( -1.000000000000000000, 0.000000000000000000, 0.000000000000000000 ) ) ;
#1171=ORIENTED_EDGE ( 'NONE', *, *, #3645, .F. ) ;
#1173=CARTESIAN_POINT ( 'NONE',  ( 9.086997423426605991, 11.58116666691846852, 38.17633527770230017 ) ) ;
#1174=CARTESIAN_POINT ( 'NONE',  ( 9.999999999999998224, -4.166666666666706931, 23.00000000000000000 ) ) ;
#1177=CARTESIAN_POINT ( 'NONE',  ( -10.70751606408958700, -3.531709963121627105, 28.15279306126447523 ) ) ;
#1181=AXIS2_PLACEMENT_3D ( 'NONE', #102, #4254, #5793 ) ;
#1182=CARTESIAN_POINT ( 'NONE',  ( 8.963566061094550008, 5.819383256046893216, 22.99383858586042351 ) ) ;
#1186=CARTESIAN_POINT ( 'NONE',  ( -9.000000000000005329, 8.999999999988014920, 23.06137295785748265 ) ) ;
#1189=LINE ( 'NONE', #3046, #1580 ) ;
#1191=CARTESIAN_POINT ( 'NONE',  ( -0.9833031778629336417, -13.77854189090673742, 35.81030296219173437 ) ) ;
#1203=CARTESIAN_POINT ( 'NONE',  ( 8.539139919159236314, 9.793760812180218878, 27.99841606626185353 ) ) ;
#1204=CARTESIAN_POINT ( 'NONE',  ( 12.35760627049921823, -9.696021465980074083, 38.00000000000000000 ) ) ;
#1205=PLANE ( 'NONE',  #3442 ) ;
#1208=CARTESIAN_POINT ( 'NONE',  ( -11.58281169573755953, 3.645573174172184405, 30.69674159737795449 ) ) ;
#1212=CARTESIAN_POINT ( 'NONE',  ( 9.793778397576030414, 8.539045536263008884, 27.99842134739334654 ) ) ;
#1213=ORIENTED_EDGE ( 'NONE', *, *, #2517, .T. ) ;
#1214=CARTESIAN_POINT ( 'NONE',  ( -6.666666666666638541, 9.999999999999998224, 23.00000000000000000 ) ) ;
#1215=LINE ( 'NONE', #5487, #3074 ) ;
#1216=CARTESIAN_POINT ( 'NONE',  ( -1.968046268140571486, -13.68733454931619953, 35.80501179064255268 ) ) ;
#1221=ADVANCED_FACE ( 'NONE', ( #490 ), #3821, .T. ) ;
#1225=CARTESIAN_POINT ( 'NONE',  ( -9.999999999999998224, -1.666666666666617225, 23.00000000000000000 ) ) ;
#1230=CARTESIAN_POINT ( 'NONE',  ( 9.999999999999998224, -3.333333333333376558, 23.00000000000000000 ) ) ;
#1231=DIRECTION ( 'NONE',  ( 0.000000000000000000, -1.000000000000000000, 0.000000000000000000 ) ) ;
#1233=CARTESIAN_POINT ( 'NONE',  ( -13.33504572891042272, 3.879012780925821247, 35.78373437249953781 ) ) ;
#1236=DIRECTION ( 'NONE',  ( 0.000000000000000000, 0.000000000000000000, -1.000000000000000000 ) ) ;
#1240=CARTESIAN_POINT ( 'NONE',  ( -8.159736356077658570, -11.57174281757876955, 35.66679457777021156 ) ) ;
#1242=CARTESIAN_POINT ( 'NONE',  ( -8.999999999988011368, -9.000000000000007105, 23.06137295785747909 ) ) ;
#1245=( GEOMETRIC_REPRESENTATION_CONTEXT ( 3 ) GLOBAL_UNCERTAINTY_ASSIGNED_CONTEXT ( ( #4246 ) ) GLOBAL_UNIT_ASSIGNED_CONTEXT ( ( #1819, #3753, #10 ) ) REPRESENTATION_CONTEXT ( 'NONE', 'WORKASPACE' ) );
#1249=CARTESIAN_POINT ( 'NONE',  ( -9.999999999999998224, -5.833333333333296622, 23.00000000000000000 ) ) ;
#1253=DIRECTION ( 'NONE',  ( 0.000000000000000000, 1.000000000000000000, 0.000000000000000000 ) ) ;
#1258=ORIENTED_EDGE ( 'NONE', *, *, #4180, .F. ) ;
#1259=CARTESIAN_POINT ( 'NONE',  ( 12.41448144607148052, -6.563799387313611788, 35.72511331161844339 ) ) ;
#1261=CARTESIAN_POINT ( 'NONE',  ( -9.778265677387498300, 4.273055220303942470, 25.59105958838676997 ) ) ;
#1270=CARTESIAN_POINT ( 'NONE',  ( -9.157688896001754841, -8.975362584346067152, 22.85246612729343596 ) ) ;
#1284=CIRCLE ( 'NONE', #1976, 15.67638808697555142 ) ;
#1286=CARTESIAN_POINT ( 'NONE',  ( 10.89081796499577059, -3.519470773090535588E-14, 28.17941898721253580 ) ) ;
#1287=CARTESIAN_POINT ( 'NONE',  ( -8.964120815521452457, 3.322922547535531734, 23.06129036953744915 ) ) ;
#1289=CARTESIAN_POINT ( 'NONE',  ( -4.154428044945160714, 8.963431230391419646, 23.04275563843252783 ) ) ;
#1294=DIRECTION ( 'NONE',  ( 1.000000000000000000, -0.000000000000000000, 0.000000000000000000 ) ) ;
#1298=B_SPLINE_SURFACE_WITH_KNOTS ( 'NONE', 3, 3, ( 
 ( #5480, #752, #5039, #4056, #317, #2160, #5975 ),
 ( #785, #4498, #4563, #6000, #5536, #5446, #2098 ),
 ( #3528, #2752, #5590, #344, #1873, #904, #405 ),
 ( #928, #2345, #3245, #871, #1346, #1378, #2784 ),
 ( #3676, #4651, #3649, #4680, #3283, #3216, #3768 ),
 ( #5683, #6085, #5070, #817, #1836, #2693, #6062 ),
 ( #2281, #430, #3702, #843, #2309, #4591, #4199 ),
 ( #4235, #2219, #5187, #4110, #6032, #2810, #1289 ),
 ( #1782, #3251, #6115, #4706, #1806, #458, #5565 ),
 ( #1752, #3188, #2719, #5097, #4148, #4617, #2251 ),
 ( #374, #1315, #5123, #4173, #5156, #1968, #4369 ),
 ( #87, #562, #4810, #2441, #3831, #2936, #5810 ),
 ( #1932, #956, #4398, #2973, #1027, #5748, #4747 ),
 ( #5312, #4335, #1410, #5348, #632, #146, #5285 ),
 ( #1532, #1056, #50, #1474, #2906, #1902, #4848 ),
 ( #3372, #2027, #3926, #3310, #3866, #5218, #2842 ),
 ( #500, #4301, #2382, #5783, #599, #1504, #5253 ),
 ( #4273, #2479, #994, #2510, #25, #120, #3797 ),
 ( #3895, #5711, #3400, #2000, #3434, #1092, #4884 ),
 ( #1438, #3340, #2878, #4781, #534, #2412, #186 ),
 ( #2152, #4938, #4490, #5473, #1119, #1682, #2115 ),
 ( #5878, #689, #4516, #4430, #2061, #721, #272 ),
 ( #1173, #3062, #3119, #1595, #1203, #3092, #3491 ),
 ( #5000, #744, #3582, #4045, #243, #2625, #5966 ),
 ( #5404, #5499, #1618, #1144, #4910, #2656, #3467 ) ),
 .UNSPECIFIED., .F., .F., .F.,
 ( 4, 3, 3, 3, 3, 3, 3, 3, 4 ),
 ( 4, 3, 4 ),
 ( 0.000000000000000000, 0.1250000000000000000, 0.2500000000000000000, 0.3750000000000000000, 0.5000000000000000000, 0.6250000000000000000, 0.7500000000000000000, 0.8750000000000000000, 1.000000000000000000 ),
 ( 0.000000000000000000, 0.5087255983319458608, 1.017451196663891722 ),
 .UNSPECIFIED. ) ;
#1304=CARTESIAN_POINT ( 'NONE',  ( -9.999999999999998224, 9.999999999999998224, 23.00000000000000000 ) ) ;
#1306=CARTESIAN_POINT ( 'NONE',  ( -9.999999999999998224, 9.999999999999998224, 23.00000000000000000 ) ) ;
#1311=CARTESIAN_POINT ( 'NONE',  ( -10.37777353962637505, 10.37777353962536608, 38.05103295300745003 ) ) ;
#1312=CARTESIAN_POINT ( 'NONE',  ( 9.928243323025453648, -2.905319074912632839E-14, 25.63579099555277807 ) ) ;
#1313=CARTESIAN_POINT ( 'NONE',  ( -10.77715421822219177, 7.077172123266720405, 30.61076540981939687 ) ) ;
#1315=CARTESIAN_POINT ( 'NONE',  ( -1.968147360634808329, 13.68731696136523546, 35.80501325620552677 ) ) ;
#1324=CARTESIAN_POINT ( 'NONE',  ( -5.247549479766072444, -10.46302782743270932, 28.11481907968152427 ) ) ;
#1325=ORIENTED_EDGE ( 'NONE', *, *, #646, .T. ) ;
#1326=CARTESIAN_POINT ( 'NONE',  ( -9.999999999999998224, -9.999999999999998224, 23.00000000000000000 ) ) ;
#1328=CARTESIAN_POINT ( 'NONE',  ( 14.67638808697554964, 1.797339169375895343E-15, 205.0000000000000568 ) ) ;
#1332=CARTESIAN_POINT ( 'NONE',  ( -9.902916272933978803, 1.657983872361913358, 22.73823205004162418 ) ) ;
#1342=CARTESIAN_POINT ( 'NONE',  ( 10.78034266696900367, -2.654236408786761814, 28.16346921039841433 ) ) ;
#1346=CARTESIAN_POINT ( 'NONE',  ( -7.732441893382013376, 9.977717576970368540, 28.03187055541259198 ) ) ;
#1350=CARTESIAN_POINT ( 'NONE',  ( 8.999999999999992895, 3.000397777471232708, 23.18288458324510515 ) ) ;
#1352=CARTESIAN_POINT ( 'NONE',  ( 15.67638808697555142, 1.919803849290630886E-15, 205.0000000000000568 ) ) ;
#1355=CARTESIAN_POINT ( 'NONE',  ( 11.08488032081242380, 11.08488032081242025, 38.00000000000000000 ) ) ;
#1364=CARTESIAN_POINT ( 'NONE',  ( 13.37091851167925149, -6.070355506015043368, 38.14417062278695880 ) ) ;
#1371=EDGE_CURVE ( 'NONE', #3081, #1401, #4508, .T. ) ;
#1375=CARTESIAN_POINT ( 'NONE',  ( 13.33504572891042095, -3.879012780925821691, 35.78373437249953781 ) ) ;
#1378=CARTESIAN_POINT ( 'NONE',  ( -7.610208295502463471, 9.462636878983097688, 25.48187184588751464 ) ) ;
#1383=CARTESIAN_POINT ( 'NONE',  ( -9.166555234036119160, -10.04707028972859106, 25.36260747786040071 ) ) ;
#1388=CARTESIAN_POINT ( 'NONE',  ( 9.858401829237468661, 10.19494410001831675, 33.01259202755186095 ) ) ;
#1396=DIRECTION ( 'NONE',  ( 0.000000000000000000, 0.000000000000000000, 1.000000000000000000 ) ) ;
#1398=EDGE_CURVE ( 'NONE', #5460, #882, #4987, .T. ) ;
#1401=VERTEX_POINT ( 'NONE', #1138 ) ;
#1407=CARTESIAN_POINT ( 'NONE',  ( 10.77715421822219355, -7.077172123266713299, 30.61076540981938976 ) ) ;
#1408=EDGE_CURVE ( 'NONE', #1157, #2972, #2564, .T. ) ;
#1410=CARTESIAN_POINT ( 'NONE',  ( 0.9505942623812212444, 12.81596724893641337, 33.26667497053200151 ) ) ;
#1416=CARTESIAN_POINT ( 'NONE',  ( -9.370308598635419983, -8.432782529159780438, 25.44727941985334496 ) ) ;
#1417=CARTESIAN_POINT ( 'NONE',  ( 11.08488032081241847, -11.08488032081242380, 38.00000000000000000 ) ) ;
#1419=CARTESIAN_POINT ( 'NONE',  ( 9.590870124851306855, 9.322893336083156512, 27.95908392747358917 ) ) ;
#1421=ORIENTED_EDGE ( 'NONE', *, *, #5944, .T. ) ;
#1427=CARTESIAN_POINT ( 'NONE',  ( 4.002955306052617068, -14.21240711833874037, 38.32637886702303121 ) ) ;
#1431=LINE ( 'NONE', #5741, #4929 ) ;
#1433=DIRECTION ( 'NONE',  ( 0.07194996680737264505, 0.07194996680737218708, -0.9948097328398209926 ) ) ;
#1438=CARTESIAN_POINT ( 'NONE',  ( 6.737147714782516950, 13.11522978513662885, 38.26633100282688105 ) ) ;
#1446=CARTESIAN_POINT ( 'NONE',  ( -9.462636878983097688, -7.610208295502463471, 25.48187184588751464 ) ) ;
#1451=PRODUCT_DEFINITION_CONTEXT ( 'detailed design', #5772, 'design' ) ;
#1453=CARTESIAN_POINT ( 'NONE',  ( -10.19629538391971124, 10.19629538389110124, 35.54424335298404003 ) ) ;
#1454=LINE ( 'NONE', #4761, #3957 ) ;
#1461=CARTESIAN_POINT ( 'NONE',  ( 9.515772848102850290, -10.27564057804868725, 33.05475024408053741 ) ) ;
#1463=ORIENTED_EDGE ( 'NONE', *, *, #2933, .F. ) ;
#1465=DIRECTION ( 'NONE',  ( -1.000000000000000000, -0.000000000000000000, -0.000000000000000000 ) ) ;
#1470=CARTESIAN_POINT ( 'NONE',  ( 8.999999999999998224, -8.999999999999998224, -167.0000000000000284 ) ) ;
#1472=AXIS2_PLACEMENT_3D ( 'NONE', #3858, #1020, #4266 ) ;
#1474=CARTESIAN_POINT ( 'NONE',  ( 1.839547822007356226, 11.79779776130985880, 30.71783115363461647 ) ) ;
#1476=CARTESIAN_POINT ( 'NONE',  ( -3.333333333333289961, 9.999999999999998224, 23.00000000000000000 ) ) ;
#1477=CARTESIAN_POINT ( 'NONE',  ( -10.37777353962477278, -10.37777353962696303, 38.05103295300743582 ) ) ;
#1481=CARTESIAN_POINT ( 'NONE',  ( -10.77711034800892875, -7.077301327650769025, 30.61076202992614270 ) ) ;
#1484=CARTESIAN_POINT ( 'NONE',  ( 10.43169748385510687, -11.73806315776973719, 38.00000000000000000 ) ) ;
#1488=CARTESIAN_POINT ( 'NONE',  ( 8.930195544526858598, -11.65680117706489760, 38.09189898655662887 ) ) ;
#1493=CARTESIAN_POINT ( 'NONE',  ( 6.787634061845150946, -9.554965159330784275, 25.51646427192168787 ) ) ;
#1499=DIRECTION ( 'NONE',  ( -1.000000000000000000, 0.000000000000000000, -0.000000000000000000 ) ) ;
#1502=CARTESIAN_POINT ( 'NONE',  ( 11.39263409468387067, -7.228600378928579318, 33.15620577507543487 ) ) ;
#1504=CARTESIAN_POINT ( 'NONE',  ( 3.423848683943063964, 9.833809958618568103, 25.60794474275442667 ) ) ;
#1505=CARTESIAN_POINT ( 'NONE',  ( -0.8289898103093434889, 9.900940235153617763, 22.73823205004162773 ) ) ;
#1512=CARTESIAN_POINT ( 'NONE',  ( -9.000000000000005329, 8.999999999988014920, 23.06137295785748265 ) ) ;
#1520=DIRECTION ( 'NONE',  ( -0.07194996680737253403, -0.07194996680737229811, -0.9948097328398209926 ) ) ;
#1521=CARTESIAN_POINT ( 'NONE',  ( 6.652779355836718977, -8.964415603276487232, 22.96342386064222296 ) ) ;
#1522=ORIENTED_EDGE ( 'NONE', *, *, #2701, .T. ) ;
#1524=CARTESIAN_POINT ( 'NONE',  ( 14.67638808697554964, -1.485455082520059617E-11, 38.18288438803429585 ) ) ;
#1527=DIRECTION ( 'NONE',  ( 0.000000000000000000, 0.000000000000000000, 1.000000000000000000 ) ) ;
#1532=CARTESIAN_POINT ( 'NONE',  ( 2.035630462091352122, 14.63234267792704557, 38.34842398122203377 ) ) ;
#1533=CARTESIAN_POINT ( 'NONE',  ( 9.969668718019493170, 9.144590365090015993, 22.73823205004162418 ) ) ;
#1538=CARTESIAN_POINT ( 'NONE',  ( -10.46302782743270754, -5.247549479766034253, 28.11481907968152782 ) ) ;
#1540=ORIENTED_EDGE ( 'NONE', *, *, #3786, .T. ) ;
#1542=CARTESIAN_POINT ( 'NONE',  ( -9.981067540164714202, -9.981067540164714202, 22.73823205004162773 ) ) ;
#1545=CARTESIAN_POINT ( 'NONE',  ( 11.39256393965315439, 7.228764404800521959, 33.15620429642044797 ) ) ;
#1553=CARTESIAN_POINT ( 'NONE',  ( 8.785602912694960409, -10.67327843797380815, 33.09221060678261495 ) ) ;
#1555=ORIENTED_EDGE ( 'NONE', *, *, #3795, .F. ) ;
#1567=CARTESIAN_POINT ( 'NONE',  ( 9.902916272933978803, -1.657983872361911803, 22.73823205004162418 ) ) ;
#1568=CARTESIAN_POINT ( 'NONE',  ( -10.72018218391586686, -10.03536489533594889, 38.06196296973735826 ) ) ;
#1569=ORIENTED_EDGE ( 'NONE', *, *, #4331, .F. ) ;
#1572=CARTESIAN_POINT ( 'NONE',  ( -9.928243323025453648, -0.8581648076836896344, 25.63579099555280294 ) ) ;
#1576=CARTESIAN_POINT ( 'NONE',  ( -11.08488032081242558, -11.08488032081241847, 38.00000000000000000 ) ) ;
#1578=CARTESIAN_POINT ( 'NONE',  ( 14.63232105816060624, 2.035738251814317223, 38.34842656511671066 ) ) ;
#1580=VECTOR ( 'NONE', #1520, 1000.000000000000000 ) ;
#1584=CARTESIAN_POINT ( 'NONE',  ( -3.570559693971999302E-14, -10.89081796499577237, 28.17941898721254290 ) ) ;
#1591=CARTESIAN_POINT ( 'NONE',  ( -11.08488032081242380, -11.08488032081242025, 38.00000000000000000 ) ) ;
#1594=VERTEX_POINT ( 'NONE', #1328 ) ;
#1595=CARTESIAN_POINT ( 'NONE',  ( 8.662453428863081228, 10.23348454756166070, 30.54531259719474079 ) ) ;
#1596=CARTESIAN_POINT ( 'NONE',  ( 9.999999999999998224, -5.833333333333365900, 23.00000000000000000 ) ) ;
#1600=CARTESIAN_POINT ( 'NONE',  ( -10.89081796499577059, -0.8880320553140184092, 28.17941898721253580 ) ) ;
#1604=CARTESIAN_POINT ( 'NONE',  ( 11.71459457793454639, 6.400384853991321954, 33.18278774224378225 ) ) ;
#1608=CARTESIAN_POINT ( 'NONE',  ( -0.9193131588476529670, -11.85339260696609465, 30.72304697887226865 ) ) ;
#1611=VERTEX_POINT ( 'NONE', #1793 ) ;
#1618=CARTESIAN_POINT ( 'NONE',  ( 10.19494410001831142, 9.858401829237472214, 33.01259202755186095 ) ) ;
#1619=CARTESIAN_POINT ( 'NONE',  ( 9.999999999999998224, 1.666666666666619223, 23.00000000000000000 ) ) ;
#1621=ORIENTED_EDGE ( 'NONE', *, *, #856, .F. ) ;
#1622=CARTESIAN_POINT ( 'NONE',  ( -10.89081796499577059, 0.8880320553140812478, 28.17941898721253580 ) ) ;
#1628=CARTESIAN_POINT ( 'NONE',  ( 12.01612071878465571, 7.393143600131257820, 35.69844150329612376 ) ) ;
#1632=CARTESIAN_POINT ( 'NONE',  ( -3.000397777471226934, 9.000000000000003553, 23.18288458324517975 ) ) ;
#1636=CARTESIAN_POINT ( 'NONE',  ( 0.9833031778629115482, -13.77854189090673742, 35.81030296219173437 ) ) ;
#1639=CYLINDRICAL_SURFACE ( 'NONE', #6037, 14.67638808697554964 ) ;
#1641=CARTESIAN_POINT ( 'NONE',  ( 12.74784844746000445, 7.336363311096732787, 38.12594328983447411 ) ) ;
#1654=VERTEX_POINT ( 'NONE', #1037 ) ;
#1657=CARTESIAN_POINT ( 'NONE',  ( -8.965668681055127820, -0.8304760625348956982, 23.09216300389307719 ) ) ;
#1667=CARTESIAN_POINT ( 'NONE',  ( -9.981067540164714202, 9.981067540164714202, 22.73823205004162418 ) ) ;
#1670=AXIS2_PLACEMENT_3D ( 'NONE', #654, #3955, #4880 ) ;
#1671=CARTESIAN_POINT ( 'NONE',  ( -3.019346778933469366, -14.42236408824967775, 38.33740271606986738 ) ) ;
#1673=LINE ( 'NONE', #2079, #587 ) ;
#1680=EDGE_CURVE ( 'NONE', #1401, #5045, #2859, .T. ) ;
#1682=CARTESIAN_POINT ( 'NONE',  ( 6.787591074359449195, 9.554964866038103466, 25.51646829178083564 ) ) ;
#1683=CARTESIAN_POINT ( 'NONE',  ( 9.939337621248920840, 6.642184745761413822, 22.73823205004162418 ) ) ;
#1687=CARTESIAN_POINT ( 'NONE',  ( -10.59950146047779640, 4.399209358691972049, 28.13666863833445220 ) ) ;
#1693=CARTESIAN_POINT ( 'NONE',  ( -5.809855716632613465, 9.930636381741159369, 22.73823205004162418 ) ) ;
#1697=CARTESIAN_POINT ( 'NONE',  ( -8.999999999999992895, -3.000397777471252692, 23.18288458324513357 ) ) ;
#1700=LINE ( 'NONE', #3142, #293 ) ;
#1707=CARTESIAN_POINT ( 'NONE',  ( -5.161660887237596640, 13.74708875321003809, 38.15586426248332685 ) ) ;
#1711=CARTESIAN_POINT ( 'NONE',  ( 12.74242197681752664, -1.902388932222474294, 33.26151580524049933 ) ) ;
#1712=CARTESIAN_POINT ( 'NONE',  ( -10.27564057804868725, 9.515772848102853843, 33.05475024408053031 ) ) ;
#1718=CARTESIAN_POINT ( 'NONE',  ( -10.43169748385510509, 11.73806315776973719, 38.00000000000000000 ) ) ;
#1720=CARTESIAN_POINT ( 'NONE',  ( -10.04707028972858929, -9.166555234036120936, 25.36260747786040426 ) ) ;
#1727=MECHANICAL_DESIGN_GEOMETRIC_PRESENTATION_REPRESENTATION('',(#59),#1245);
#1731=CARTESIAN_POINT ( 'NONE',  ( 9.999999999999998224, -9.999999999999998224, 23.00000000000000000 ) ) ;
#1732=CARTESIAN_POINT ( 'NONE',  ( -11.08488032081241670, 11.08488032081242558, 38.00000000000000000 ) ) ;
#1741=B_SPLINE_SURFACE_WITH_KNOTS ( 'NONE', 3, 1, ( 
 ( #929, #4707, #1667 ),
 ( #1718, #3623, #3567 ),
 ( #4064, #5511, #5485 ),
 ( #5981, #1214, #3105 ),
 ( #2641, #4536, #1693 ),
 ( #2511, #4399, #4748 ),
 ( #4336, #1476, #996 ),
 ( #3798, #3373, #1028 ),
 ( #1057, #26, #1505 ),
 ( #2843, #502, #4782 ),
 ( #147, #3341, #4885 ),
 ( #2383, #2907, #2937 ),
 ( #5254, #4849, #2413 ),
 ( #633, #2879, #5712 ),
 ( #5286, #4275, #535 ),
 ( #4811, #5784, #2028 ),
 ( #2001, #4302, #5749 ),
 ( #51, #1903, #3435 ) ),
 .UNSPECIFIED., .F., .F., .F.,
 ( 4, 2, 2, 2, 2, 2, 2, 2, 4 ),
 ( 2, 1, 2 ),
 ( 0.000000000000000000, 0.1250000000000000000, 0.2500000000000000000, 0.3750000000000000000, 0.5000000000000000000, 0.6250000000000000000, 0.7500000000000000000, 0.8750000000000000000, 1.000000000000000000 ),
 ( 0.000000000000000000, 1.000000000000000000, 1.017451196663891722 ),
 .UNSPECIFIED. ) ;
#1744=( NAMED_UNIT ( * ) SI_UNIT ( $, .STERADIAN. ) SOLID_ANGLE_UNIT ( ) );
#1746=CARTESIAN_POINT ( 'NONE',  ( 14.74111653287706147, -1.016991241531516321, 38.35393095385146012 ) ) ;
#1749=CARTESIAN_POINT ( 'NONE',  ( -12.01622299351614309, 7.392961014695935695, 35.69843844696172397 ) ) ;
#1752=CARTESIAN_POINT ( 'NONE',  ( -3.019346778933468478, 14.42236408824967420, 38.33740271606986738 ) ) ;
#1755=CLOSED_SHELL ( 'NONE', ( #903, #4378, #5152, #5023, #3116, #2355, #1040, #8, #56, #3308, #5561, #716, #3389, #3785, #6031, #779, #1221, #4832, #3079, #2136, #2856, #2241 ) ) ;
#1770=CARTESIAN_POINT ( 'NONE',  ( -9.999999999999998224, 9.166666666666673180, 23.00000000000000000 ) ) ;
#1772=CARTESIAN_POINT ( 'NONE',  ( 9.557272410707515320, -9.557272410707506438, 28.03893107092314452 ) ) ;
#1773=EDGE_LOOP ( 'NONE', ( #761, #3241, #2703, #1540, #624, #6019 ) ) ;
#1776=CARTESIAN_POINT ( 'NONE',  ( 10.37777353962571425, 10.37777353962603044, 38.05103295300744293 ) ) ;
#1778=CARTESIAN_POINT ( 'NONE',  ( 12.45811160333930623, -3.759380242563083119, 33.24069127598784235 ) ) ;
#1780=CARTESIAN_POINT ( 'NONE',  ( -11.02055295301484428, 6.248212340465905790, 30.63787875916901626 ) ) ;
#1782=CARTESIAN_POINT ( 'NONE',  ( -4.002955306052619733, 14.21240711833874037, 38.32637886702303121 ) ) ;
#1789=CARTESIAN_POINT ( 'NONE',  ( -6.563799387313615341, -12.41448144607147874, 35.72511331161845050 ) ) ;
#1793=CARTESIAN_POINT ( 'NONE',  ( 8.999999999988068211, 9.000000000000005329, 23.06137295785747554 ) ) ;
#1796=CARTESIAN_POINT ( 'NONE',  ( -9.999999999999998224, 0.8333333333333826642, 23.00000000000000000 ) ) ;
#1797=DIRECTION ( 'NONE',  ( 0.000000000000000000, -1.000000000000000000, -0.000000000000000000 ) ) ;
#1802=( LENGTH_UNIT ( ) NAMED_UNIT ( * ) SI_UNIT ( .MILLI., .METRE. ) );
#1803=CARTESIAN_POINT ( 'NONE',  ( 9.833809958618568103, -3.423848683943063964, 25.60794474275442667 ) ) ;
#1806=CARTESIAN_POINT ( 'NONE',  ( -3.531709963121634210, 10.70751606408959411, 28.15279306126448233 ) ) ;
#1811=CARTESIAN_POINT ( 'NONE',  ( -11.06391443747533998, 9.691632641776340762, 38.07293523736174023 ) ) ;
#1812=CARTESIAN_POINT ( 'NONE',  ( -10.08321815271041544, -9.378998278013590095, 27.91486726096250948 ) ) ;
#1818=DIRECTION ( 'NONE',  ( -0.000000000000000000, -0.000000000000000000, -1.000000000000000000 ) ) ;
#1819=( LENGTH_UNIT ( ) NAMED_UNIT ( * ) SI_UNIT ( .MILLI., .METRE. ) );
#1821=CARTESIAN_POINT ( 'NONE',  ( -9.981067540164714202, 9.981067540164714202, 22.73823205004162418 ) ) ;
#1831=CARTESIAN_POINT ( 'NONE',  ( 12.74411457810409232, -5.685785403169735019, 35.74643938915853880 ) ) ;
#1832=CARTESIAN_POINT ( 'NONE',  ( -8.975362584346067152, 9.157688896001753065, 22.85246612729342885 ) ) ;
#1836=CARTESIAN_POINT ( 'NONE',  ( -6.095798759547075285, 10.32656711695237561, 28.09297316833070468 ) ) ;
#1845=CARTESIAN_POINT ( 'NONE',  ( -14.20502198335936050, 3.811938596482205011, 38.16892149784423793 ) ) ;
#1848=CARTESIAN_POINT ( 'NONE',  ( 8.983694681928700021, 9.994658916190591214, 22.80938439471025703 ) ) ;
#1863=VERTEX_POINT ( 'NONE', #5361 ) ;
#1870=CARTESIAN_POINT ( 'NONE',  ( 9.370308891928093686, -8.432825516645548802, 25.44727539999419719 ) ) ;
#1873=CARTESIAN_POINT ( 'NONE',  ( -8.539045536263005332, 9.793778397576030414, 27.99842134739334654 ) ) ;
#1878=CARTESIAN_POINT ( 'NONE',  ( -9.858401829237470437, -10.19494410001831497, 33.01259202755186095 ) ) ;
#1879=CARTESIAN_POINT ( 'NONE',  ( 9.999999999999998224, -9.999999999999998224, 23.00000000000000000 ) ) ;
#1881=DIRECTION ( 'NONE',  ( 0.000000000000000000, 0.000000000000000000, -1.000000000000000000 ) ) ;
#1882=CARTESIAN_POINT ( 'NONE',  ( -6.075059976385840166, -13.36876581604936653, 38.14410695834219922 ) ) ;
#1886=DIRECTION ( 'NONE',  ( 0.000000000000000000, 0.000000000000000000, -1.000000000000000000 ) ) ;
#1889=CARTESIAN_POINT ( 'NONE',  ( 4.666802875123989836, -12.24718835365691127, 33.22501703466258505 ) ) ;
#1891=ORIENTED_EDGE ( 'NONE', *, *, #1162, .T. ) ;
#1901=EDGE_CURVE ( 'NONE', #1611, #5798, #4236, .T. ) ;
#1902=CARTESIAN_POINT ( 'NONE',  ( 1.716658579843636012, 9.908812303639313868, 25.63028407385522911 ) ) ;
#1903=CARTESIAN_POINT ( 'NONE',  ( 9.999999999999998224, 9.999999999999998224, 23.00000000000000000 ) ) ;
#1904=CARTESIAN_POINT ( 'NONE',  ( -14.18603054855838508, -3.792815487222209736, 38.16899780669729125 ) ) ;
#1907=CARTESIAN_POINT ( 'NONE',  ( -8.970286642449650572, -8.321944142006522327, 22.89273687632151066 ) ) ;
#1916=CARTESIAN_POINT ( 'NONE',  ( 14.48620990986883506, -2.403201876585592256, 38.17751351274289817 ) ) ;
#1917=CARTESIAN_POINT ( 'NONE',  ( 10.08321815271041899, -9.378998278013591872, 27.91486726096250948 ) ) ;
#1919=B_SPLINE_CURVE_WITH_KNOTS ( 'NONE', 3,
 ( #1512, #1034, #31, #5229, #1453, #2886 ),
 .UNSPECIFIED., .F., .F.,
 ( 4, 2, 4 ),
 ( 0.003149728260038243185, 0.01070802693369690868, 0.01826632560735557548 ),
 .UNSPECIFIED. ) ;
#1922=DIRECTION ( 'NONE',  ( 0.000000000000000000, 0.000000000000000000, -1.000000000000000000 ) ) ;
#1926=CARTESIAN_POINT ( 'NONE',  ( 9.378998278013590095, -10.08321815271041721, 27.91486726096250948 ) ) ;
#1932=CARTESIAN_POINT ( 'NONE',  ( 7.589415207398531038E-16, 14.74111653287705792, 38.35393095385146012 ) ) ;
#1934=CARTESIAN_POINT ( 'NONE',  ( -11.65565333135050885, -8.931668428568697138, 38.09186409098167303 ) ) ;
#1942=CARTESIAN_POINT ( 'NONE',  ( -8.967351122863068014, -7.487361748921619764, 22.92808036848186504 ) ) ;
#1948=CARTESIAN_POINT ( 'NONE',  ( 3.000397777471251359, -9.000000000000000000, 23.18288458324515133 ) ) ;
#1949=CARTESIAN_POINT ( 'NONE',  ( 3.314202382262465996, -14.30535051437892768, 38.17196567842750454 ) ) ;
#1950=VERTEX_POINT ( 'NONE', #1352 ) ;
#1956=CARTESIAN_POINT ( 'NONE',  ( 10.04707028972859106, -9.166555234036120936, 25.36260747786040426 ) ) ;
#1964=CARTESIAN_POINT ( 'NONE',  ( 11.57174281757876599, -8.159736356077656794, 35.66679457777021156 ) ) ;
#1967=ORIENTED_EDGE ( 'NONE', *, *, #2969, .T. ) ;
#1968=CARTESIAN_POINT ( 'NONE',  ( -1.716690548177159714, 9.908812100099982700, 25.63028262842344773 ) ) ;
#1969=AXIS2_PLACEMENT_3D ( 'NONE', #4704, #1025, #2904 ) ;
#1971=CARTESIAN_POINT ( 'NONE',  ( -11.94400843721153116, -8.542271628753789869, 38.10037361971537706 ) ) ;
#1976=AXIS2_PLACEMENT_3D ( 'NONE', #5330, #5800, #1159 ) ;
#1978=CARTESIAN_POINT ( 'NONE',  ( 9.144590365090015993, -9.969668718019493170, 22.73823205004162773 ) ) ;
#1979=EDGE_CURVE ( 'NONE', #5045, #3083, #5130, .T. ) ;
#1980=CARTESIAN_POINT ( 'NONE',  ( -8.999999999988011368, -9.000000000000007105, 23.06137295785747909 ) ) ;
#1981=LINE ( 'NONE', #3905, #3847 ) ;
#1989=CARTESIAN_POINT ( 'NONE',  ( 5.685785403169718144, -12.74411457810409765, 35.74643938915854591 ) ) ;
#1997=CARTESIAN_POINT ( 'NONE',  ( 8.999999999999998224, 8.999999999999998224, -167.0000000000000284 ) ) ;
#2000=CARTESIAN_POINT ( 'NONE',  ( 5.390571672161876826, 11.22195964661421819, 30.65936073406735218 ) ) ;
#2001=CARTESIAN_POINT ( 'NONE',  ( 10.43169748385510864, 11.73806315776973896, 38.00000000000000711 ) ) ;
#2002=CARTESIAN_POINT ( 'NONE',  ( -11.04414289254774140, -9.677595944629031166, 38.07286884698770280 ) ) ;
#2005=CARTESIAN_POINT ( 'NONE',  ( -10.85317354580219273, 1.776706711792239046, 28.17414650202874427 ) ) ;
#2007=CARTESIAN_POINT ( 'NONE',  ( 6.666666666666638541, -9.999999999999998224, 23.00000000000000000 ) ) ;
#2009=CARTESIAN_POINT ( 'NONE',  ( 8.967351122863068014, 7.487361748921619764, 22.92808036848186504 ) ) ;
#2010=CARTESIAN_POINT ( 'NONE',  ( -2.411881101062222310, -14.48475173028215401, 38.17746263717076971 ) ) ;
#2018=CARTESIAN_POINT ( 'NONE',  ( 8.926329112024040668, -11.12736491637287806, 35.63514765224429937 ) ) ;
#2021=CARTESIAN_POINT ( 'NONE',  ( 0.000000000000000000, 8.999999999999998224, -167.0000000000000284 ) ) ;
#2022=CARTESIAN_POINT ( 'NONE',  ( -15.67638808697555142, 0.000000000000000000, 205.0000000000000568 ) ) ;
#2027=CARTESIAN_POINT ( 'NONE',  ( 2.923529524533198032, 13.51119013911331024, 35.79437308157104525 ) ) ;
#2028=CARTESIAN_POINT ( 'NONE',  ( 8.309552794738978676, 9.958856949317492990, 22.73823205004162418 ) ) ;
#2033=CARTESIAN_POINT ( 'NONE',  ( -9.871311131128940985, -2.570253631893256951, 25.61911440830482789 ) ) ;
#2035=ORIENTED_EDGE ( 'NONE', *, *, #3794, .F. ) ;
#2037=CARTESIAN_POINT ( 'NONE',  ( -1.657983872361911803, -9.902916272933980579, 22.73823205004162773 ) ) ;
#2039=AXIS2_PLACEMENT_3D ( 'NONE', #2815, #3680, #4241 ) ;
#2040=CARTESIAN_POINT ( 'NONE',  ( 9.977717576970368540, 7.732441893382015152, 28.03187055541259198 ) ) ;
#2042=CIRCLE ( 'NONE', #2447, 15.67638808697555142 ) ;
#2049=CARTESIAN_POINT ( 'NONE',  ( 0.8581648076836596584, -9.928243323025412792, 25.63579099555278873 ) ) ;
#2052=PLANE ( 'NONE',  #2150 ) ;
#2057=CARTESIAN_POINT ( 'NONE',  ( -9.306281718482047438, -9.306281718482059873, 25.54332486258996582 ) ) ;
#2061=CARTESIAN_POINT ( 'NONE',  ( 7.732441893382044462, 9.977717576970368540, 28.03187055541259909 ) ) ;
#2062=CARTESIAN_POINT ( 'NONE',  ( 15.56315586465741774, 2.164213882025733504, 38.00000000000000711 ) ) ;
#2067=CARTESIAN_POINT ( 'NONE',  ( -13.50805179034378867, -5.845970755595367940, 38.28811402100271977 ) ) ;
#2070=CARTESIAN_POINT ( 'NONE',  ( 0.8289898103093435999, -9.900940235153619540, 22.73823205004163128 ) ) ;
#2072=CARTESIAN_POINT ( 'NONE',  ( 13.11530391916999605, 6.736970939972929173, 38.26632377370044935 ) ) ;
#2075=EDGE_LOOP ( 'NONE', ( #3887, #5515, #2421, #4317 ) ) ;
#2077=CARTESIAN_POINT ( 'NONE',  ( -1.839547822007357114, -11.79779776130985880, 30.71783115363462002 ) ) ;
#2079=CARTESIAN_POINT ( 'NONE',  ( -14.67638808697554964, 0.000000000000000000, 205.0000000000000568 ) ) ;
#2092=DIRECTION ( 'NONE',  ( 0.000000000000000000, -0.000000000000000000, -1.000000000000000000 ) ) ;
#2096=CARTESIAN_POINT ( 'NONE',  ( -11.85339260696609287, -0.9193131588476038951, 30.72304697887226510 ) ) ;
#2098=CARTESIAN_POINT ( 'NONE',  ( -9.157688896001733525, 8.975362584346067152, 22.85246612729342885 ) ) ;
#2103=CARTESIAN_POINT ( 'NONE',  ( -3.879012780925823467, -13.33504572891042272, 35.78373437249953781 ) ) ;
#2104=ORIENTED_EDGE ( 'NONE', *, *, #181, .T. ) ;
#2115=CARTESIAN_POINT ( 'NONE',  ( 6.652784304366590185, 8.964415574088988592, 22.96342341013486887 ) ) ;
#2116=CARTESIAN_POINT ( 'NONE',  ( 11.08488032081241670, -11.08488032081242558, 38.00000000000000000 ) ) ;
#2122=CARTESIAN_POINT ( 'NONE',  ( -9.638809746143360613, -5.954763795926145242, 25.54536317066256501 ) ) ;
#2129=CARTESIAN_POINT ( 'NONE',  ( 11.22195964661421641, 5.390571672161841299, 30.65936073406735574 ) ) ;
#2136=ADVANCED_FACE ( 'NONE', ( #5224 ), #4078, .F. ) ;
#2137=CARTESIAN_POINT ( 'NONE',  ( 2.570253631893271606, -9.871311131128953420, 25.61911440830483144 ) ) ;
#2150=AXIS2_PLACEMENT_3D ( 'NONE', #5869, #5396, #1136 ) ;
#2152=CARTESIAN_POINT ( 'NONE',  ( 7.570044180282069490, 12.64059746256323002, 38.23931193745811186 ) ) ;
#2155=CARTESIAN_POINT ( 'NONE',  ( -9.999999999999998224, 8.999999999999998224, 23.00000000000000000 ) ) ;
#2158=CARTESIAN_POINT ( 'NONE',  ( -9.370308891928093686, 8.432825516645547026, 25.44727539999419719 ) ) ;
#2160=CARTESIAN_POINT ( 'NONE',  ( -10.04707028972859106, 9.166555234036119160, 25.36260747786040071 ) ) ;
#2163=AXIS2_PLACEMENT_3D ( 'NONE', #2233, #2767, #4133 ) ;
#2175=CARTESIAN_POINT ( 'NONE',  ( 1.776762854451772622, -10.85316926984840968, 28.17414535953234278 ) ) ;
#2189=CARTESIAN_POINT ( 'NONE',  ( 9.999999999999998224, -0.8333333333333816650, 23.00000000000000000 ) ) ;
#2192=CARTESIAN_POINT ( 'NONE',  ( 9.708537589994000072, -5.113933401365548193, 25.56820946177495557 ) ) ;
#2193=CARTESIAN_POINT ( 'NONE',  ( -8.963431154120575783, 4.154433491267528922, 23.04275521548131067 ) ) ;
#2196=B_SPLINE_SURFACE_WITH_KNOTS ( 'NONE', 3, 1, ( 
 ( #1591, #3489, #5402 ),
 ( #5022, #5144, #770 ),
 ( #888, #6049, #4670 ),
 ( #420, #4549, #2235 ),
 ( #333, #1249, #5519 ),
 ( #2769, #2652, #4189 ),
 ( #857, #3146, #4639 ),
 ( #2209, #1225, #5553 ),
 ( #5111, #4163, #5056 ),
 ( #4100, #1796, #4581 ),
 ( #2736, #304, #1332 ),
 ( #5580, #805, #6016 ),
 ( #4073, #5991, #359 ),
 ( #3237, #834, #2709 ),
 ( #2682, #388, #2269 ),
 ( #6075, #3693, #5605 ),
 ( #2298, #1770, #6104 ),
 ( #1732, #1306, #1821 ) ),
 .UNSPECIFIED., .F., .F., .F.,
 ( 4, 2, 2, 2, 2, 2, 2, 2, 4 ),
 ( 2, 1, 2 ),
 ( 0.000000000000000000, 0.1250000000000000833, 0.2500000000000001665, 0.3750000000000001110, 0.5000000000000001110, 0.6250000000000001110, 0.7500000000000000000, 0.8750000000000000000, 1.000000000000000000 ),
 ( 0.000000000000000000, 1.000000000000000000, 1.017451196663891722 ),
 .UNSPECIFIED. ) ;
#2199=EDGE_LOOP ( 'NONE', ( #3949, #5614, #2647, #1055 ) ) ;
#2201=CARTESIAN_POINT ( 'NONE',  ( -7.610208295502499887, -9.462636878983104793, 25.48187184588751819 ) ) ;
#2206=CARTESIAN_POINT ( 'NONE',  ( -8.999999999999998224, -9.999999999999998224, 23.00000000000000000 ) ) ;
#2209=CARTESIAN_POINT ( 'NONE',  ( -15.56315586465741951, -2.164213882025732172, 38.00000000000000711 ) ) ;
#2216=CARTESIAN_POINT ( 'NONE',  ( 11.58281169573755953, -3.645573174172184405, 30.69674159737795449 ) ) ;
#2217=CARTESIAN_POINT ( 'NONE',  ( -9.708537589994000072, 5.113933401365539311, 25.56820946177495557 ) ) ;
#2219=CARTESIAN_POINT ( 'NONE',  ( -4.807938790076510926, 13.07368784376655491, 35.76776929191790089 ) ) ;
#2224=AXIS2_PLACEMENT_3D ( 'NONE', #4077, #5993, #6022 ) ;
#2225=CARTESIAN_POINT ( 'NONE',  ( -10.19494410001831142, -9.858401829237470437, 33.01259202755186095 ) ) ;
#2226=ORIENTED_EDGE ( 'NONE', *, *, #605, .T. ) ;
#2231=VECTOR ( 'NONE', #5962, 1000.000000000000000 ) ;
#2233=CARTESIAN_POINT ( 'NONE',  ( 0.000000000000000000, 0.000000000000000000, 205.0000000000000568 ) ) ;
#2235=CARTESIAN_POINT ( 'NONE',  ( -9.939337621248920840, -6.642184745761411158, 22.73823205004162418 ) ) ;
#2241=ADVANCED_FACE ( 'NONE', ( #5049 ), #1639, .F. ) ;
#2247=CARTESIAN_POINT ( 'NONE',  ( 9.871311131128940985, -2.570253631893350210, 25.61911440830482789 ) ) ;
#2248=CARTESIAN_POINT ( 'NONE',  ( -12.60026679007841466, 2.830884587392776819, 33.25110354061416018 ) ) ;
#2250=EDGE_CURVE ( 'NONE', #1863, #4386, #1673, .T. ) ;
#2251=CARTESIAN_POINT ( 'NONE',  ( -2.491918585145397991, 8.964680801521355491, 23.07363600708416129 ) ) ;
#2255=CARTESIAN_POINT ( 'NONE',  ( 0.000000000000000000, -8.999999999999998224, -167.0000000000000284 ) ) ;
#2260=CARTESIAN_POINT ( 'NONE',  ( -5.533593864557681208, -11.98089146579572883, 33.20390238845318009 ) ) ;
#2262=LINE ( 'NONE', #1326, #3361 ) ;
#2264=ORIENTED_EDGE ( 'NONE', *, *, #2594, .F. ) ;
#2269=CARTESIAN_POINT ( 'NONE',  ( -9.939337621248920840, 6.642184745761469777, 22.73823205004162418 ) ) ;
#2275=CARTESIAN_POINT ( 'NONE',  ( 9.692295192625326905, 11.06325188662640180, 38.07291408809467015 ) ) ;
#2277=CARTESIAN_POINT ( 'NONE',  ( 10.89081796499577237, -0.8880320553140826911, 28.17941898721253580 ) ) ;
#2279=CARTESIAN_POINT ( 'NONE',  ( -8.965240787521256749, 1.660914622755444991, 23.08598164463087343 ) ) ;
#2281=CARTESIAN_POINT ( 'NONE',  ( -5.845970755595359947, 13.50805179034379044, 38.28811402100272687 ) ) ;
#2289=CARTESIAN_POINT ( 'NONE',  ( -9.632247231687292910, -10.63625351335941716, 35.59852902770369809 ) ) ;
#2294=DIRECTION ( 'NONE',  ( 0.000000000000000000, 0.000000000000000000, 1.000000000000000000 ) ) ;
#2297=VERTEX_POINT ( 'NONE', #4928 ) ;
#2298=CARTESIAN_POINT ( 'NONE',  ( -11.73806315776973364, 10.43169748385510864, 38.00000000000000000 ) ) ;
#2304=CARTESIAN_POINT ( 'NONE',  ( 8.952355667640917503, 11.66870637430316648, 38.09164563373214918 ) ) ;
#2306=CARTESIAN_POINT ( 'NONE',  ( 13.77854189090673742, -1.299091064715344294E-14, 35.81030296219172726 ) ) ;
#2309=CARTESIAN_POINT ( 'NONE',  ( -5.247549479766024483, 10.46302782743270754, 28.11481907968152427 ) ) ;
#2314=B_SPLINE_CURVE_WITH_KNOTS ( 'NONE', 3,
 ( #3882, #4869, #619, #1350, #820, #2315 ),
 .UNSPECIFIED., .F., .F.,
 ( 4, 2, 4 ),
 ( 0.002357188415687185273, 0.01135824717474477781, 0.02035930593380236991 ),
 .UNSPECIFIED. ) ;
#2315=CARTESIAN_POINT ( 'NONE',  ( 8.999999999988068211, 9.000000000000005329, 23.06137295785747554 ) ) ;
#2317=CARTESIAN_POINT ( 'NONE',  ( -14.67638808697555319, 1.484446970801598990E-11, 38.18288438803429585 ) ) ;
#2320=ORIENTED_EDGE ( 'NONE', *, *, #1162, .F. ) ;
#2323=DIRECTION ( 'NONE',  ( 0.000000000000000000, -1.000000000000000000, 0.000000000000000000 ) ) ;
#2325=LINE ( 'NONE', #2860, #6047 ) ;
#2339=CARTESIAN_POINT ( 'NONE',  ( 9.306281718482082965, 9.306281718482070531, 25.54332486258998358 ) ) ;
#2344=ORIENTED_EDGE ( 'NONE', *, *, #5176, .T. ) ;
#2345=CARTESIAN_POINT ( 'NONE',  ( -8.159736356077649688, 11.57174281757876777, 35.66679457777021867 ) ) ;
#2352=EDGE_CURVE ( 'NONE', #5798, #4467, #5363, .T. ) ;
#2353=CARTESIAN_POINT ( 'NONE',  ( -12.11088206474084572, -8.328520801854336852, 38.20782360758019536 ) ) ;
#2355=ADVANCED_FACE ( 'NONE', ( #172 ), #2052, .F. ) ;
#2363=CIRCLE ( 'NONE', #5859, 15.67638808697555142 ) ;
#2366=CARTESIAN_POINT ( 'NONE',  ( 13.16326790094642263, -6.508032323544555631, 38.13839276770974607 ) ) ;
#2369=CARTESIAN_POINT ( 'NONE',  ( 8.007183658747738519, -11.03292118881348394, 33.12420745160152791 ) ) ;
#2374=CARTESIAN_POINT ( 'NONE',  ( -8.999999999999998224, -8.999999999999998224, 23.00000000000000000 ) ) ;
#2379=CARTESIAN_POINT ( 'NONE',  ( 11.12726264164139245, -8.926511697459380557, 35.63515070857870626 ) ) ;
#2380=AXIS2_PLACEMENT_3D ( 'NONE', #180, #2966, #3461 ) ;
#2382=CARTESIAN_POINT ( 'NONE',  ( 3.759380242563083563, 12.45811160333930800, 33.24069127598783524 ) ) ;
#2383=CARTESIAN_POINT ( 'NONE',  ( 4.260267006495017661, 15.12434353048566749, 38.00000000000000711 ) ) ;
#2386=EDGE_LOOP ( 'NONE', ( #2104, #664, #3640, #119 ) ) ;
#2389=B_SPLINE_CURVE_WITH_KNOTS ( 'NONE', 3,
 ( #1980, #2854, #5792, #1948, #3, #4760 ),
 .UNSPECIFIED., .F., .F.,
 ( 4, 2, 4 ),
 ( 0.002357188415687252060, 0.01135824717474482638, 0.02035930593380240114 ),
 .UNSPECIFIED. ) ;
#2390=CARTESIAN_POINT ( 'NONE',  ( -11.66987820548587074, 8.950926204225673644, 38.09167945787530840 ) ) ;
#2391=CARTESIAN_POINT ( 'NONE',  ( 10.63625351335941893, 9.632247231687287581, 35.59852902770369099 ) ) ;
#2395=FACE_OUTER_BOUND ( 'NONE', #4321, .T. ) ;
#2401=CARTESIAN_POINT ( 'NONE',  ( 3.531709963121631102, -10.70751606408959589, 28.15279306126448589 ) ) ;
#2410=CARTESIAN_POINT ( 'NONE',  ( 9.269614772507654976, -9.245260337044141963, 25.40693856330804223 ) ) ;
#2412=CARTESIAN_POINT ( 'NONE',  ( 5.954811582427137040, 9.638809502600501844, 25.54535933516314117 ) ) ;
#2413=CARTESIAN_POINT ( 'NONE',  ( 4.147343260682193389, 9.916251082295017838, 22.73823205004162418 ) ) ;
#2417=CARTESIAN_POINT ( 'NONE',  ( -9.378998278013590095, -10.08321815271042432, 27.91486726096250948 ) ) ;
#2418=CARTESIAN_POINT ( 'NONE',  ( -3.333333333333376558, -9.999999999999998224, 23.00000000000000000 ) ) ;
#2421=ORIENTED_EDGE ( 'NONE', *, *, #2558, .T. ) ;
#2422=CARTESIAN_POINT ( 'NONE',  ( 10.37777353962571425, 10.37777353962603044, 38.05103295300744293 ) ) ;
#2425=CARTESIAN_POINT ( 'NONE',  ( 14.20502198335932142, -3.811938596482332020, 38.16892149784424504 ) ) ;
#2426=CARTESIAN_POINT ( 'NONE',  ( 3.423816715609377948, -9.833810162157929469, 25.60794618818621515 ) ) ;
#2428=EDGE_LOOP ( 'NONE', ( #955, #1026, #4159, #2226, #6103, #1463 ) ) ;
#2436=CARTESIAN_POINT ( 'NONE',  ( 8.967351122863068014, -7.487361748921665061, 22.92808036848186504 ) ) ;
#2441=CARTESIAN_POINT ( 'NONE',  ( -0.9193131588476050053, 11.85339260696609642, 30.72304697887226510 ) ) ;
#2447=AXIS2_PLACEMENT_3D ( 'NONE', #5062, #3991, #2539 ) ;
#2451=CARTESIAN_POINT ( 'NONE',  ( 5.273949241992675674, -14.79903580929012463, 38.00000000000000711 ) ) ;
#2456=CARTESIAN_POINT ( 'NONE',  ( -9.692295192624374778, -11.06325188662722248, 38.07291408809469857 ) ) ;
#2465=CARTESIAN_POINT ( 'NONE',  ( 6.563632016262921809, -12.41454131244164216, 35.72510948639917672 ) ) ;
#2475=CARTESIAN_POINT ( 'NONE',  ( 8.963566137365393871, -5.819377809724670669, 22.99383900881164067 ) ) ;
#2476=VECTOR ( 'NONE', #541, 1000.000000000000000 ) ;
#2479=CARTESIAN_POINT ( 'NONE',  ( 4.807771419025856474, 13.07374771013670767, 35.76776546669863421 ) ) ;
#2482=CARTESIAN_POINT ( 'NONE',  ( 9.999999999999998224, 9.999999999999998224, 23.00000000000000000 ) ) ;
#2483=CARTESIAN_POINT ( 'NONE',  ( -14.67638808697651420, -0.9595328539162122361, 38.18288438803428875 ) ) ;
#2485=ORIENTED_EDGE ( 'NONE', *, *, #6093, .F. ) ;
#2488=CARTESIAN_POINT ( 'NONE',  ( -8.963566061094550008, -5.819383256046894992, 22.99383858586043061 ) ) ;
#2490=CARTESIAN_POINT ( 'NONE',  ( -9.999999999999998224, -9.999999999999998224, 23.00000000000000000 ) ) ;
#2492=CARTESIAN_POINT ( 'NONE',  ( 9.618700053625529378, 10.13908112636437231, 30.46372964425718521 ) ) ;
#2499=CARTESIAN_POINT ( 'NONE',  ( 7.610208295502465248, -9.462636878983104793, 25.48187184588751819 ) ) ;
#2500=VERTEX_POINT ( 'NONE', #6128 ) ;
#2506=CARTESIAN_POINT ( 'NONE',  ( -9.557272410707509991, -9.557272410707509991, 28.03893107092312675 ) ) ;
#2510=CARTESIAN_POINT ( 'NONE',  ( 4.532931003857846086, 11.42336634021359387, 30.68084270896568810 ) ) ;
#2511=CARTESIAN_POINT ( 'NONE',  ( -5.273949241992676562, 14.79903580929012286, 38.00000000000000711 ) ) ;
#2515=CARTESIAN_POINT ( 'NONE',  ( -11.22195964661421641, -5.390571672161848404, 30.65936073406735574 ) ) ;
#2517=EDGE_CURVE ( 'NONE', #3083, #3081, #5082, .T. ) ;
#2519=CARTESIAN_POINT ( 'NONE',  ( 8.333333333333316162, -9.999999999999998224, 23.00000000000000000 ) ) ;
#2521=CARTESIAN_POINT ( 'NONE',  ( 9.871311131128940985, 2.570253631893256951, 25.61911440830482789 ) ) ;
#2527=CARTESIAN_POINT ( 'NONE',  ( 2.923529524533178936, -13.51119013911330846, 35.79437308157104525 ) ) ;
#2529=VERTEX_POINT ( 'NONE', #353 ) ;
#2531=CARTESIAN_POINT ( 'NONE',  ( 13.19705249345142484, 6.492124056756818362, 38.13875458540265129 ) ) ;
#2534=CARTESIAN_POINT ( 'NONE',  ( -8.999999999988011368, -9.000000000000007105, 23.06137295785747909 ) ) ;
#2539=DIRECTION ( 'NONE',  ( 1.000000000000000000, 0.000000000000000000, 0.000000000000000000 ) ) ;
#2543=CARTESIAN_POINT ( 'NONE',  ( -10.85316926984840791, -1.776762854451772622, 28.17414535953233923 ) ) ;
#2546=CARTESIAN_POINT ( 'NONE',  ( -0.8333333333333816650, -9.999999999999998224, 23.00000000000000000 ) ) ;
#2551=EDGE_CURVE ( 'NONE', #3749, #2972, #2262, .T. ) ;
#2552=CARTESIAN_POINT ( 'NONE',  ( 11.79778917763282209, 1.839621235173125369, 30.71783072571432882 ) ) ;
#2558=EDGE_CURVE ( 'NONE', #3160, #3083, #1981, .T. ) ;
#2560=CARTESIAN_POINT ( 'NONE',  ( -1.016991241531519652, -14.74111653287705792, 38.35393095385146012 ) ) ;
#2564=LINE ( 'NONE', #1084, #6051 ) ;
#2573=CARTESIAN_POINT ( 'NONE',  ( 13.97471987708211216, -7.178663235509287865, 38.00000000000000000 ) ) ;
#2576=CARTESIAN_POINT ( 'NONE',  ( -13.77854189090673742, 0.9833031778629290898, 35.81030296219172726 ) ) ;
#2582=CARTESIAN_POINT ( 'NONE',  ( 10.70751606408959411, 3.531709963121627105, 28.15279306126448944 ) ) ;
#2588=CARTESIAN_POINT ( 'NONE',  ( -1.660914622755444991, -8.965240787521260302, 23.08598164463088054 ) ) ;
#2592=CARTESIAN_POINT ( 'NONE',  ( 10.37777353962571425, 10.37777353962603044, 38.05103295300744293 ) ) ;
#2593=EDGE_CURVE ( 'NONE', #1594, #5460, #1454, .T. ) ;
#2594=EDGE_CURVE ( 'NONE', #251, #2529, #2819, .T. ) ;
#2602=CARTESIAN_POINT ( 'NONE',  ( 15.12434353048566749, 4.260267006495017661, 38.00000000000001421 ) ) ;
#2606=CARTESIAN_POINT ( 'NONE',  ( -12.45812449473958239, -3.759289558891018679, 33.24069098933199484 ) ) ;
#2608=EDGE_CURVE ( 'NONE', #1863, #1594, #4151, .T. ) ;
#2610=CARTESIAN_POINT ( 'NONE',  ( 12.74411457810409232, 5.685785403169719032, 35.74643938915853880 ) ) ;
#2614=B_SPLINE_CURVE_WITH_KNOTS ( 'NONE', 3,
 ( #3774, #1811, #2390, #5194, #5131, #3708, #5690, #3682, #1845, #5102, #908, #846, #437, #2317 ),
 .UNSPECIFIED., .F., .F.,
 ( 4, 2, 2, 2, 2, 2, 4 ),
 ( 8.673617379884035472E-18, 0.002860246893306399221, 0.004290370339959594277, 0.005720493786612789767, 0.008580740679919178146, 0.01001086412657237017, 0.01144098757322556392 ),
 .UNSPECIFIED. ) ;
#2615=CARTESIAN_POINT ( 'NONE',  ( -4.154433491267528034, -8.963431154120577560, 23.04275521548131778 ) ) ;
#2625=CARTESIAN_POINT ( 'NONE',  ( 9.245260337044141963, 9.269614772507654976, 25.40693856330804223 ) ) ;
#2626=CARTESIAN_POINT ( 'NONE',  ( 9.910574073276151807, -3.317157231508649495, 22.73823205004162418 ) ) ;
#2627=CARTESIAN_POINT ( 'NONE',  ( 0.000000000000000000, 0.000000000000000000, 38.00000000000000000 ) ) ;
#2632=CARTESIAN_POINT ( 'NONE',  ( -10.23348454756166070, 8.662453428863081228, 30.54531259719474079 ) ) ;
#2641=CARTESIAN_POINT ( 'NONE',  ( -7.178663235509282536, 13.97471987708211216, 38.00000000000000000 ) ) ;
#2643=CARTESIAN_POINT ( 'NONE',  ( 0.9193131588475976779, -11.85339260696609465, 30.72304697887227576 ) ) ;
#2647=ORIENTED_EDGE ( 'NONE', *, *, #2551, .T. ) ;
#2649=LINE ( 'NONE', #1304, #498 ) ;
#2652=CARTESIAN_POINT ( 'NONE',  ( -9.999999999999998224, -4.166666666666622554, 23.00000000000000000 ) ) ;
#2655=LINE ( 'NONE', #6107, #195 ) ;
#2656=CARTESIAN_POINT ( 'NONE',  ( 10.04707028972858929, 9.166555234036119160, 25.36260747786040071 ) ) ;
#2657=CARTESIAN_POINT ( 'NONE',  ( 13.97471987708211216, 7.178663235509286089, 38.00000000000000000 ) ) ;
#2662=CARTESIAN_POINT ( 'NONE',  ( -13.90087379555095204, 4.954793796408211826, 38.30989703917856559 ) ) ;
#2666=CIRCLE ( 'NONE', #3843, 15.67638808697555142 ) ;
#2675=CARTESIAN_POINT ( 'NONE',  ( -4.986905650496099796, -8.963498645742987492, 23.01829711214648455 ) ) ;
#2682=CARTESIAN_POINT ( 'NONE',  ( -13.47611570251764768, 8.069545871843430973, 38.00000000000000000 ) ) ;
#2689=CARTESIAN_POINT ( 'NONE',  ( 11.02055295301484428, -6.248212340465907566, 30.63787875916901626 ) ) ;
#2691=CARTESIAN_POINT ( 'NONE',  ( -9.977717576970368540, 7.732441893382045350, 28.03187055541259909 ) ) ;
#2693=CARTESIAN_POINT ( 'NONE',  ( -5.954763795926128367, 9.638809746143360613, 25.54536317066255791 ) ) ;
#2701=EDGE_CURVE ( 'NONE', #5813, #3749, #6076, .T. ) ;
#2702=CARTESIAN_POINT ( 'NONE',  ( -5.819377809724670669, -8.963566137365395647, 22.99383900881164777 ) ) ;
#2703=ORIENTED_EDGE ( 'NONE', *, *, #2933, .T. ) ;
#2709=CARTESIAN_POINT ( 'NONE',  ( -9.930636381741159369, 5.809855716632678302, 22.73823205004162418 ) ) ;
#2715=CARTESIAN_POINT ( 'NONE',  ( 7.356224370874624441, 12.70872189800938834, 38.12480727770459055 ) ) ;
#2716=CARTESIAN_POINT ( 'NONE',  ( 12.81596724893641159, 0.9505942623811802772, 33.26667497053200151 ) ) ;
#2717=CARTESIAN_POINT ( 'NONE',  ( -13.07374771013671122, 4.807771419025852033, 35.76776546669862711 ) ) ;
#2719=CARTESIAN_POINT ( 'NONE',  ( -2.830884587392748841, 12.60026679007841288, 33.25110354061416018 ) ) ;
#2726=CARTESIAN_POINT ( 'NONE',  ( -15.67638808697555142, 0.000000000000000000, 205.0000000000000568 ) ) ;
#2736=CARTESIAN_POINT ( 'NONE',  ( -15.56315586465742484, 2.164213882025736613, 38.00000000000000711 ) ) ;
#2741=FACE_OUTER_BOUND ( 'NONE', #5238, .T. ) ;
#2744=CARTESIAN_POINT ( 'NONE',  ( -1.900794651634388321, 14.58443831393954859, 38.18056006088393417 ) ) ;
#2746=EDGE_CURVE ( 'NONE', #2529, #3160, #176, .T. ) ;
#2749=CARTESIAN_POINT ( 'NONE',  ( 11.85339260696609287, -2.780846643040693260E-14, 30.72304697887226510 ) ) ;
#2750=CARTESIAN_POINT ( 'NONE',  ( -12.11088206474084750, 8.328520801854340405, 38.20782360758020957 ) ) ;
#2752=CARTESIAN_POINT ( 'NONE',  ( -8.926329112024045997, 11.12736491637288339, 35.63514765224430647 ) ) ;
#2761=CARTESIAN_POINT ( 'NONE',  ( -6.925743867604849946, -10.16167434176052176, 28.06532504456334820 ) ) ;
#2767=DIRECTION ( 'NONE',  ( -0.000000000000000000, -0.000000000000000000, -1.000000000000000000 ) ) ;
#2769=CARTESIAN_POINT ( 'NONE',  ( -14.79903580929011930, -5.273949241992674786, 38.00000000000000000 ) ) ;
#2777=CARTESIAN_POINT ( 'NONE',  ( -4.709709529607297718, 13.90855959397112862, 38.16103891068026144 ) ) ;
#2779=CARTESIAN_POINT ( 'NONE',  ( 8.965240827029074211, 1.660911000355770328, 23.08598180255751942 ) ) ;
#2784=CARTESIAN_POINT ( 'NONE',  ( -7.487361748921619764, 8.967351122863068014, 22.92808036848186504 ) ) ;
#2787=FACE_OUTER_BOUND ( 'NONE', #2428, .T. ) ;
#2789=CARTESIAN_POINT ( 'NONE',  ( -11.02058084744346544, -6.248091806769219048, 30.63788045528724524 ) ) ;
#2791=CARTESIAN_POINT ( 'NONE',  ( -7.869812776064898152, -10.50531938289192979, 30.57803900350706883 ) ) ;
#2792=ORIENTED_EDGE ( 'NONE', *, *, #1051, .T. ) ;
#2805=CARTESIAN_POINT ( 'NONE',  ( 0.9766276285328842066, 14.65181115585160931, 38.18271774125523876 ) ) ;
#2808=PLANE ( 'NONE',  #1969 ) ;
#2810=CARTESIAN_POINT ( 'NONE',  ( -4.273103006804785053, 9.778265433844637755, 25.59105575288735324 ) ) ;
#2815=CARTESIAN_POINT ( 'NONE',  ( 0.000000000000000000, 0.000000000000000000, 205.0000000000000568 ) ) ;
#2819=B_SPLINE_CURVE_WITH_KNOTS ( 'NONE', 3,
 ( #2951, #2456, #3353, #1008, #4311, #3319, #1882, #1035, #64, #2010, #5725, #5693, #2887, #131, #3807, #1949, #5822, #515, #973, #3777, #4789, #5763, #1488, #542, #4347, #4863 ),
 .UNSPECIFIED., .F., .F.,
 ( 4, 2, 2, 2, 2, 2, 2, 2, 2, 2, 2, 2, 4 ),
 ( 2.453269466693398698E-18, 0.002857484983890242261, 0.004286227475835359922, 0.005714969967780478451, 0.008572454951670712905, 0.01000119744361583143, 0.01142993993556095170, 0.01428742491945118875, 0.01571616741139630902, 0.01714490990334142928, 0.02000239488723166634, 0.02143113737917678660, 0.02285987987112190686 ),
 .UNSPECIFIED. ) ;
#2820=CARTESIAN_POINT ( 'NONE',  ( 9.933255351449997050, 9.419333092093003401, 30.50691708577705796 ) ) ;
#2830=CARTESIAN_POINT ( 'NONE',  ( 4.986905650496026077, -8.963498645742987492, 23.01829711214648455 ) ) ;
#2839=CARTESIAN_POINT ( 'NONE',  ( 12.64059746256322470, -7.570044180282070378, 38.23931193745811186 ) ) ;
#2842=CARTESIAN_POINT ( 'NONE',  ( 2.491918585145488585, 8.964680801521355491, 23.07363600708416129 ) ) ;
#2843=CARTESIAN_POINT ( 'NONE',  ( 1.082228759108216032, 15.67638808697554786, 38.00000000000000711 ) ) ;
#2854=CARTESIAN_POINT ( 'NONE',  ( -6.000548030722248072, -9.000000000000003553, 23.13502304888920591 ) ) ;
#2855=AXIS2_PLACEMENT_3D ( 'NONE', #423, #1253, #4642 ) ;
#2856=ADVANCED_FACE ( 'NONE', ( #5146 ), #3135, .F. ) ;
#2858=ORIENTED_EDGE ( 'NONE', *, *, #3786, .F. ) ;
#2859=LINE ( 'NONE', #4257, #866 ) ;
#2860=CARTESIAN_POINT ( 'NONE',  ( -10.54244016040621013, 10.54244016040621013, 30.50000000000000000 ) ) ;
#2864=CARTESIAN_POINT ( 'NONE',  ( 14.67638808697506292, -0.4806947631990224901, 38.18288438803429585 ) ) ;
#2866=CARTESIAN_POINT ( 'NONE',  ( 3.645499761006324224, -11.58282027941459269, 30.69674202529824569 ) ) ;
#2867=ORIENTED_EDGE ( 'NONE', *, *, #2558, .F. ) ;
#2868=VERTEX_POINT ( 'NONE', #1355 ) ;
#2873=AXIS2_PLACEMENT_3D ( 'NONE', #3298, #1396, #3325 ) ;
#2878=CARTESIAN_POINT ( 'NONE',  ( 6.400535080091637852, 11.71455171164206988, 33.18278799730942552 ) ) ;
#2879=CARTESIAN_POINT ( 'NONE',  ( 5.833333333333365900, 9.999999999999998224, 23.00000000000000000 ) ) ;
#2883=CARTESIAN_POINT ( 'NONE',  ( -11.39256393965315439, -7.228764404800518406, 33.15620429642044087 ) ) ;
#2886=CARTESIAN_POINT ( 'NONE',  ( -10.37777353962637505, 10.37777353962536608, 38.05103295300745003 ) ) ;
#2887=CARTESIAN_POINT ( 'NONE',  ( -0.4914066504967060656, -14.67601930163249513, 38.18288424882399568 ) ) ;
#2893=CARTESIAN_POINT ( 'NONE',  ( 11.06391443747510195, -9.691632641776605439, 38.07293523736169760 ) ) ;
#2894=CARTESIAN_POINT ( 'NONE',  ( 7.570233152424892253, -12.64046943599297101, 38.23931941266578605 ) ) ;
#2904=DIRECTION ( 'NONE',  ( 0.000000000000000000, -0.000000000000000000, -1.000000000000000000 ) ) ;
#2906=CARTESIAN_POINT ( 'NONE',  ( 1.776706711792238824, 10.85317354580219451, 28.17414650202874427 ) ) ;
#2907=CARTESIAN_POINT ( 'NONE',  ( 3.333333333333376558, 9.999999999999998224, 23.00000000000000000 ) ) ;
#2908=CARTESIAN_POINT ( 'NONE',  ( -14.67638808697555319, 1.484446970801598990E-11, 38.18288438803429585 ) ) ;
#2911=CARTESIAN_POINT ( 'NONE',  ( -8.964415603276487232, -6.652779355836718089, 22.96342386064221941 ) ) ;
#2912=CARTESIAN_POINT ( 'NONE',  ( 7.178663235509283425, -13.97471987708211572, 38.00000000000000000 ) ) ;
#2914=DIRECTION ( 'NONE',  ( 1.000000000000000000, 0.000000000000000000, -0.000000000000000000 ) ) ;
#2918=ORIENTED_EDGE ( 'NONE', *, *, #4180, .T. ) ;
#2920=CARTESIAN_POINT ( 'NONE',  ( 8.159736356077644359, -11.57174281757876599, 35.66679457777021156 ) ) ;
#2921=ORIENTED_EDGE ( 'NONE', *, *, #3607, .T. ) ;
#2922=CARTESIAN_POINT ( 'NONE',  ( -9.618700053625529378, 10.13908112636436520, 30.46372964425718521 ) ) ;
#2924=ORIENTED_EDGE ( 'NONE', *, *, #3415, .T. ) ;
#2931=CARTESIAN_POINT ( 'NONE',  ( 10.67320828294309543, -8.785766938566929696, 33.09220912812762805 ) ) ;
#2933=EDGE_CURVE ( 'NONE', #464, #6095, #5104, .T. ) ;
#2936=CARTESIAN_POINT ( 'NONE',  ( -0.8581648076837100625, 9.928243323025455425, 25.63579099555274965 ) ) ;
#2937=CARTESIAN_POINT ( 'NONE',  ( 3.317157231508649495, 9.910574073276151807, 22.73823205004162418 ) ) ;
#2941=ORIENTED_EDGE ( 'NONE', *, *, #2746, .T. ) ;
#2945=CARTESIAN_POINT ( 'NONE',  ( -11.79779776130985702, 1.839547822007354894, 30.71783115363461647 ) ) ;
#2947=CARTESIAN_POINT ( 'NONE',  ( -5.833333333333365900, -9.999999999999998224, 23.00000000000000000 ) ) ;
#2950=LINE ( 'NONE', #1070, #3169 ) ;
#2951=CARTESIAN_POINT ( 'NONE',  ( -10.37777353962477278, -10.37777353962696303, 38.05103295300743582 ) ) ;
#2959=CARTESIAN_POINT ( 'NONE',  ( 10.27356722921338594, -10.12138240269939082, 35.55812462721154787 ) ) ;
#2966=DIRECTION ( 'NONE',  ( -1.000000000000000000, 0.000000000000000000, 0.000000000000000000 ) ) ;
#2969=EDGE_CURVE ( 'NONE', #5798, #2297, #1919, .T. ) ;
#2972=VERTEX_POINT ( 'NONE', #3806 ) ;
#2973=CARTESIAN_POINT ( 'NONE',  ( 2.334726591726390495E-14, 11.85339260696609465, 30.72304697887226510 ) ) ;
#2980=CARTESIAN_POINT ( 'NONE',  ( -8.964680801521355491, -2.491918585145397991, 23.07363600708416129 ) ) ;
#2982=CARTESIAN_POINT ( 'NONE',  ( 6.642184745761413822, -9.939337621248920840, 22.73823205004162773 ) ) ;
#2984=CARTESIAN_POINT ( 'NONE',  ( 11.69030472852370650, 2.742560498089724685, 30.70728637550628903 ) ) ;
#2990=CARTESIAN_POINT ( 'NONE',  ( -4.954793796408214490, -13.90087379555094493, 38.30989703917857270 ) ) ;
#3001=CARTESIAN_POINT ( 'NONE',  ( 9.916251082295017838, 4.147343260682109900, 22.73823205004162418 ) ) ;
#3004=EDGE_LOOP ( 'NONE', ( #3016, #1621 ) ) ;
#3006=CARTESIAN_POINT ( 'NONE',  ( -14.42236408824967064, -3.019346778933471143, 38.33740271606986028 ) ) ;
#3008=CARTESIAN_POINT ( 'NONE',  ( -10.43169748385511042, -11.73806315776973541, 38.00000000000000711 ) ) ;
#3010=CARTESIAN_POINT ( 'NONE',  ( 12.41454131244163506, 6.563632016262926250, 35.72510948639917672 ) ) ;
#3013=EDGE_CURVE ( 'NONE', #1611, #3081, #2950, .T. ) ;
#3015=CARTESIAN_POINT ( 'NONE',  ( -4.399209358691967608, -10.59950146047779818, 28.13666863833443799 ) ) ;
#3016=ORIENTED_EDGE ( 'NONE', *, *, #2608, .F. ) ;
#3019=CARTESIAN_POINT ( 'NONE',  ( 13.74495680931392450, 5.167291852657578843, 38.15579506865712034 ) ) ;
#3032=CARTESIAN_POINT ( 'NONE',  ( -11.85339260696609287, 2.318493676985545998E-14, 30.72304697887226510 ) ) ;
#3039=EDGE_CURVE ( 'NONE', #4467, #3160, #2389, .T. ) ;
#3041=CARTESIAN_POINT ( 'NONE',  ( 12.60026679007841288, 2.830884587392749285, 33.25110354061416018 ) ) ;
#3046=CARTESIAN_POINT ( 'NONE',  ( 10.54244016040621190, 10.54244016040621013, 30.50000000000000000 ) ) ;
#3048=CARTESIAN_POINT ( 'NONE',  ( -0.8581648076837764538, -9.928243323025448319, 25.63579099555280294 ) ) ;
#3050=DIRECTION ( 'NONE',  ( -0.000000000000000000, -0.000000000000000000, -1.000000000000000000 ) ) ;
#3059=ORIENTED_EDGE ( 'NONE', *, *, #3039, .F. ) ;
#3062=CARTESIAN_POINT ( 'NONE',  ( 8.926511697459378780, 11.12726264164139600, 35.63515070857870626 ) ) ;
#3063=CARTESIAN_POINT ( 'NONE',  ( 9.969668718019493170, -9.144590365090033757, 22.73823205004162418 ) ) ;
#3066=ORIENTED_EDGE ( 'NONE', *, *, #2701, .F. ) ;
#3069=CARTESIAN_POINT ( 'NONE',  ( -14.63234267792704735, 2.035630462091347237, 38.34842398122203377 ) ) ;
#3074=VECTOR ( 'NONE', #3106, 1000.000000000000000 ) ;
#3075=CARTESIAN_POINT ( 'NONE',  ( 9.370308598635419983, 8.432782529159778662, 25.44727941985334496 ) ) ;
#3077=ORIENTED_EDGE ( 'NONE', *, *, #668, .T. ) ;
#3079=ADVANCED_FACE ( 'NONE', ( #4861 ), #5538, .F. ) ;
#3080=CARTESIAN_POINT ( 'NONE',  ( -2.491918585145488585, -8.964680801521357267, 23.07363600708416840 ) ) ;
#3081=VERTEX_POINT ( 'NONE', #1997 ) ;
#3083=VERTEX_POINT ( 'NONE', #1470 ) ;
#3092=CARTESIAN_POINT ( 'NONE',  ( 8.432825516645548802, 9.370308891928093686, 25.44727539999419719 ) ) ;
#3098=CARTESIAN_POINT ( 'NONE',  ( -11.58116666691846852, 9.086997423426605991, 38.17633527770230017 ) ) ;
#3102=CARTESIAN_POINT ( 'NONE',  ( 8.970286642449650572, 8.321944142006520551, 22.89273687632151066 ) ) ;
#3105=CARTESIAN_POINT ( 'NONE',  ( -6.642184745761413822, 9.939337621248920840, 22.73823205004162418 ) ) ;
#3106=DIRECTION ( 'NONE',  ( -1.000000000000000000, -0.000000000000000000, -0.000000000000000000 ) ) ;
#3107=CARTESIAN_POINT ( 'NONE',  ( -1.902388932222473850, -12.74242197681752486, 33.26151580524049223 ) ) ;
#3116=ADVANCED_FACE ( 'NONE', ( #5283 ), #2808, .F. ) ;
#3119=CARTESIAN_POINT ( 'NONE',  ( 8.785766938566926143, 10.67320828294310076, 33.09220912812762094 ) ) ;
#3124=CARTESIAN_POINT ( 'NONE',  ( -13.11522978513662885, 6.737147714782517838, 38.26633100282688815 ) ) ;
#3133=CARTESIAN_POINT ( 'NONE',  ( 9.999999999999998224, -9.999999999999998224, -167.0000000000000284 ) ) ;
#3135=B_SPLINE_SURFACE_WITH_KNOTS ( 'NONE', 3, 3, ( 
 ( #3816, #2959, #5832, #3390, #1917, #1956, #5275 ),
 ( #4829, #5735, #1461, #4798, #5331, #523, #3362 ),
 ( #3912, #2018, #1553, #3853, #5204, #944, #3884 ),
 ( #137, #2920, #2369, #4290, #4356, #2499, #5802 ),
 ( #2894, #1016, #5771, #586, #109, #1493, #1521 ),
 ( #5302, #2465, #3419, #4771, #5700, #39, #1079 ),
 ( #1044, #1989, #486, #4872, #621, #4388, #2830 ),
 ( #548, #4733, #1889, #4263, #3784, #5241, #14 ),
 ( #1427, #3326, #983, #2866, #2401, #2426, #4319 ),
 ( #74, #2527, #294, #647, #4986, #2137, #4539 ),
 ( #3569, #5420, #3482, #4417, #2175, #1111, #5983 ),
 ( #168, #1636, #4956, #2643, #203, #2049, #5892 ),
 ( #4449, #711, #4066, #1134, #1584, #3946, #1160 ),
 ( #2560, #1191, #4034, #1608, #5488, #3048, #5953 ),
 ( #3506, #1216, #3107, #2077, #3541, #3976, #2588 ),
 ( #1671, #4899, #3454, #4478, #5459, #5014, #3080 ),
 ( #231, #2103, #760, #4925, #4003, #5920, #5368 ),
 ( #2990, #733, #5866, #5394, #3015, #676, #2615 ),
 ( #4504, #259, #2260, #5545, #1324, #5512, #2675 ),
 ( #325, #1789, #3685, #3136, #5047, #5080, #2702 ),
 ( #3626, #5166, #795, #3711, #2761, #3261, #4662 ),
 ( #3226, #1240, #4572, #2791, #5597, #2201, #826 ),
 ( #909, #412, #6006, #5573, #351, #4156, #5134 ),
 ( #4630, #2289, #4092, #380, #879, #4181, #1270 ),
 ( #4599, #6094, #2225, #6068, #1812, #1720, #5627 ) ),
 .UNSPECIFIED., .F., .F., .F.,
 ( 4, 3, 3, 3, 3, 3, 3, 3, 4 ),
 ( 4, 3, 4 ),
 ( 0.000000000000000000, 0.1250000000000000000, 0.2500000000000000000, 0.3750000000000000000, 0.5000000000000000000, 0.6250000000000000000, 0.7500000000000000000, 0.8750000000000000000, 1.000000000000000000 ),
 ( 0.000000000000000000, 0.5087255983319457497, 1.017451196663891499 ),
 .UNSPECIFIED. ) ;
#3136=CARTESIAN_POINT ( 'NONE',  ( -6.248212340465907566, -11.02055295301484428, 30.63787875916901626 ) ) ;
#3142=CARTESIAN_POINT ( 'NONE',  ( -9.999999999999998224, -9.999999999999998224, -167.0000000000000284 ) ) ;
#3146=CARTESIAN_POINT ( 'NONE',  ( -9.999999999999998224, -3.333333333333286408, 23.00000000000000000 ) ) ;
#3157=CARTESIAN_POINT ( 'NONE',  ( 8.965668681055126044, -0.8304760625349946190, 23.09216300389308074 ) ) ;
#3159=CARTESIAN_POINT ( 'NONE',  ( -8.964680801521355491, 2.491918585145488141, 23.07363600708416129 ) ) ;
#3160=VERTEX_POINT ( 'NONE', #4011 ) ;
#3169=VECTOR ( 'NONE', #1881, 1000.000000000000000 ) ;
#3178=LINE ( 'NONE', #1731, #2231 ) ;
#3184=CARTESIAN_POINT ( 'NONE',  ( -10.03503361918909143, 10.72051346006269235, 38.06197354439402147 ) ) ;
#3185=CARTESIAN_POINT ( 'NONE',  ( 14.74111653287705792, -5.477421655106639269E-15, 38.35393095385146012 ) ) ;
#3186=CARTESIAN_POINT ( 'NONE',  ( -12.45811160333930623, 3.759380242563082675, 33.24069127598783524 ) ) ;
#3188=CARTESIAN_POINT ( 'NONE',  ( -2.923529524533181601, 13.51119013911330846, 35.79437308157104525 ) ) ;
#3189=EDGE_CURVE ( 'NONE', #464, #1950, #5764, .T. ) ;
#3191=PRODUCT_DEFINITION_SHAPE ( 'NONE', 'NONE',  #118 ) ;
#3208=ORIENTED_EDGE ( 'NONE', *, *, #822, .F. ) ;
#3209=CARTESIAN_POINT ( 'NONE',  ( 11.08488032081242025, -11.08488032081242203, 38.00000000000000711 ) ) ;
#3213=CARTESIAN_POINT ( 'NONE',  ( 14.21238549857230815, -4.003063095775586611, 38.32638145091770809 ) ) ;
#3214=CARTESIAN_POINT ( 'NONE',  ( -10.16167434176051465, 6.925743867604855275, 28.06532504456334465 ) ) ;
#3215=EDGE_LOOP ( 'NONE', ( #4128, #450, #5530, #240, #4109, #5631 ) ) ;
#3216=CARTESIAN_POINT ( 'NONE',  ( -6.787634061845148281, 9.554965159330777169, 25.51646427192168431 ) ) ;
#3226=CARTESIAN_POINT ( 'NONE',  ( -8.328520801854340405, -12.11088206474084927, 38.20782360758020246 ) ) ;
#3227=ORIENTED_EDGE ( 'NONE', *, *, #2352, .T. ) ;
#3237=CARTESIAN_POINT ( 'NONE',  ( -13.97471987708211216, 7.178663235509287865, 38.00000000000000711 ) ) ;
#3241=ORIENTED_EDGE ( 'NONE', *, *, #3189, .F. ) ;
#3245=CARTESIAN_POINT ( 'NONE',  ( -8.007183658747742072, 11.03292118881348394, 33.12420745160152791 ) ) ;
#3248=CARTESIAN_POINT ( 'NONE',  ( 10.59950146047779462, -4.399209358691971161, 28.13666863833444154 ) ) ;
#3251=CARTESIAN_POINT ( 'NONE',  ( -3.878911688431554428, 13.33506331686138147, 35.78373290693656372 ) ) ;
#3253=ORIENTED_EDGE ( 'NONE', *, *, #2608, .T. ) ;
#3259=VECTOR ( 'NONE', #1797, 1000.000000000000000 ) ;
#3261=CARTESIAN_POINT ( 'NONE',  ( -6.787591074359450971, -9.554964866038112348, 25.51646829178083919 ) ) ;
#3269=CARTESIAN_POINT ( 'NONE',  ( 14.65251043020005461, -0.9663357036150953538, 38.18273246053423975 ) ) ;
#3271=CARTESIAN_POINT ( 'NONE',  ( 9.306281718482058096, -9.306281718482106058, 25.54332486258998358 ) ) ;
#3279=CARTESIAN_POINT ( 'NONE',  ( 13.90087379555094671, -4.954793796408218043, 38.30989703917857270 ) ) ;
#3283=CARTESIAN_POINT ( 'NONE',  ( -6.925838250501022308, 10.16165675636470489, 28.06531976343183743 ) ) ;
#3285=CARTESIAN_POINT ( 'NONE',  ( -9.000000000000005329, 8.999999999988014920, 23.06137295785748265 ) ) ;
#3288=CARTESIAN_POINT ( 'NONE',  ( -9.590870124851305079, -9.322893336083154736, 27.95908392747358207 ) ) ;
#3293=ORIENTED_EDGE ( 'NONE', *, *, #1408, .T. ) ;
#3295=DIRECTION ( 'NONE',  ( 0.000000000000000000, 1.000000000000000000, -0.000000000000000000 ) ) ;
#3296=LINE ( 'NONE', #5272, #5228 ) ;
#3298=CARTESIAN_POINT ( 'NONE',  ( 0.000000000000000000, 0.000000000000000000, 205.0000000000000568 ) ) ;
#3300=VERTEX_POINT ( 'NONE', #1116 ) ;
#3304=CARTESIAN_POINT ( 'NONE',  ( 0.000000000000000000, 0.000000000000000000, 0.000000000000000000 ) ) ;
#3305=CARTESIAN_POINT ( 'NONE',  ( 9.557272410707515320, 9.557272410707515320, 28.03893107092314096 ) ) ;
#3306=CARTESIAN_POINT ( 'NONE',  ( 10.16167434176051820, -6.925743867604847281, 28.06532504456334109 ) ) ;
#3308=ADVANCED_FACE ( 'NONE', ( #5875 ), #2196, .T. ) ;
#3310=CARTESIAN_POINT ( 'NONE',  ( 2.742560498089770427, 11.69030472852371005, 30.70728637550628548 ) ) ;
#3311=CARTESIAN_POINT ( 'NONE',  ( 12.35760627049922533, 9.696021465980072307, 37.99999999999999289 ) ) ;
#3314=CARTESIAN_POINT ( 'NONE',  ( -8.999999999988011368, -9.000000000000007105, 23.06137295785747909 ) ) ;
#3318=CARTESIAN_POINT ( 'NONE',  ( 11.12736491637288516, 8.926329112024047774, 35.63514765224430647 ) ) ;
#3319=CARTESIAN_POINT ( 'NONE',  ( -6.512188664276555627, -13.16119478149536270, 38.13833290264207676 ) ) ;
#3325=DIRECTION ( 'NONE',  ( 1.000000000000000000, 0.000000000000000000, -0.000000000000000000 ) ) ;
#3326=CARTESIAN_POINT ( 'NONE',  ( 3.878911688431552651, -13.33506331686138147, 35.78373290693656372 ) ) ;
#3340=CARTESIAN_POINT ( 'NONE',  ( 6.563799387313611788, 12.41448144607148230, 35.72511331161844339 ) ) ;
#3341=CARTESIAN_POINT ( 'NONE',  ( 1.666666666666713814, 9.999999999999998224, 23.00000000000000000 ) ) ;
#3348=CARTESIAN_POINT ( 'NONE',  ( -12.64046943599296924, -7.570233152424897582, 38.23931941266577894 ) ) ;
#3349=CARTESIAN_POINT ( 'NONE',  ( -6.642184745761470666, -9.939337621248920840, 22.73823205004162773 ) ) ;
#3353=CARTESIAN_POINT ( 'NONE',  ( -8.952355667639968928, -11.66870637430388591, 38.09164563373219181 ) ) ;
#3361=VECTOR ( 'NONE', #2914, 1000.000000000000000 ) ;
#3362=CARTESIAN_POINT ( 'NONE',  ( 9.157688896001733525, -8.975362584346067152, 22.85246612729343596 ) ) ;
#3369=CARTESIAN_POINT ( 'NONE',  ( -10.54244016040621190, -10.54244016040621013, 30.50000000000000000 ) ) ;
#3370=CARTESIAN_POINT ( 'NONE',  ( 9.462636878983097688, -7.610208295502498999, 25.48187184588751464 ) ) ;
#3372=CARTESIAN_POINT ( 'NONE',  ( 3.019346778933469810, 14.42236408824967775, 38.33740271606986738 ) ) ;
#3373=CARTESIAN_POINT ( 'NONE',  ( -1.666666666666619223, 9.999999999999998224, 23.00000000000000000 ) ) ;
#3377=CARTESIAN_POINT ( 'NONE',  ( -9.554965159330777169, -6.787634061845147393, 25.51646427192168431 ) ) ;
#3378=CARTESIAN_POINT ( 'NONE',  ( -0.8289898103094419657, -9.900940235153617763, 22.73823205004162773 ) ) ;
#3381=CARTESIAN_POINT ( 'NONE',  ( 9.378998278013591872, 10.08321815271042610, 27.91486726096250948 ) ) ;
#3385=CARTESIAN_POINT ( 'NONE',  ( 15.67638808697555142, 1.640158138686712206E-15, 38.00000000000000711 ) ) ;
#3389=ADVANCED_FACE ( 'NONE', ( #1014, #5239 ), #4221, .T. ) ;
#3390=CARTESIAN_POINT ( 'NONE',  ( 10.13908112636436520, -9.618700053625531154, 30.46372964425718521 ) ) ;
#3397=LINE ( 'NONE', #3369, #5373 ) ;
#3398=CARTESIAN_POINT ( 'NONE',  ( 8.964415574088988592, -6.652784304366590185, 22.96342341013486887 ) ) ;
#3400=CARTESIAN_POINT ( 'NONE',  ( 5.533593864557681208, 11.98089146579572883, 33.20390238845318009 ) ) ;
#3401=FACE_OUTER_BOUND ( 'NONE', #3517, .T. ) ;
#3405=CARTESIAN_POINT ( 'NONE',  ( -9.793778397576030414, -8.539045536263005332, 27.99842134739335009 ) ) ;
#3408=CARTESIAN_POINT ( 'NONE',  ( 1.666666666666619223, -9.999999999999998224, 23.00000000000000000 ) ) ;
#3415=EDGE_CURVE ( 'NONE', #2529, #5460, #758, .T. ) ;
#3419=CARTESIAN_POINT ( 'NONE',  ( 6.400384853991321066, -11.71459457793454995, 33.18278774224378225 ) ) ;
#3424=CARTESIAN_POINT ( 'NONE',  ( 13.90645689909075777, 4.715863500831550148, 38.16097513848706768 ) ) ;
#3428=FACE_OUTER_BOUND ( 'NONE', #3581, .T. ) ;
#3432=B_SPLINE_CURVE_WITH_KNOTS ( 'NONE', 3,
 ( #4778, #3792, #5679, #3305, #2339, #5706 ),
 .UNSPECIFIED., .F., .F.,
 ( 4, 2, 4 ),
 ( 2.991083261082871196E-05, 0.007589224902417050257, 0.01514853897222326155 ),
 .UNSPECIFIED. ) ;
#3434=CARTESIAN_POINT ( 'NONE',  ( 5.247549479766072444, 10.46302782743270932, 28.11481907968152427 ) ) ;
#3435=CARTESIAN_POINT ( 'NONE',  ( 9.981067540164714202, 9.981067540164714202, 22.73823205004162418 ) ) ;
#3442=AXIS2_PLACEMENT_3D ( 'NONE', #2155, #1231, #2092 ) ;
#3443=CARTESIAN_POINT ( 'NONE',  ( -11.79778917763282209, -1.839621235173125369, 30.71783072571432882 ) ) ;
#3447=CARTESIAN_POINT ( 'NONE',  ( 11.58282027941459091, 3.645499761006323780, 30.69674202529824925 ) ) ;
#3449=ORIENTED_EDGE ( 'NONE', *, *, #675, .T. ) ;
#3454=CARTESIAN_POINT ( 'NONE',  ( -2.830884587392779039, -12.60026679007841643, 33.25110354061416018 ) ) ;
#3461=DIRECTION ( 'NONE',  ( 0.000000000000000000, 0.000000000000000000, 1.000000000000000000 ) ) ;
#3467=CARTESIAN_POINT ( 'NONE',  ( 9.994658916190592990, 8.983694681928700021, 22.80938439471025703 ) ) ;
#3468=CARTESIAN_POINT ( 'NONE',  ( 13.47611570251764412, -8.069545871843434526, 37.99999999999999289 ) ) ;
#3473=EDGE_CURVE ( 'NONE', #4944, #1157, #1284, .T. ) ;
#3474=CARTESIAN_POINT ( 'NONE',  ( -14.74111653287705792, -1.380323371794770872E-15, 38.35393095385146012 ) ) ;
#3476=CARTESIAN_POINT ( 'NONE',  ( -7.178663235509287865, -13.97471987708211039, 38.00000000000000000 ) ) ;
#3477=CARTESIAN_POINT ( 'NONE',  ( 10.77711034800893053, 7.077301327650772578, 30.61076202992614270 ) ) ;
#3482=CARTESIAN_POINT ( 'NONE',  ( 1.902479615894475451, -12.74240908541723982, 33.26151609189631841 ) ) ;
#3489=CARTESIAN_POINT ( 'NONE',  ( -9.999999999999998224, -9.999999999999998224, 23.00000000000000000 ) ) ;
#3491=CARTESIAN_POINT ( 'NONE',  ( 8.321939193476740826, 8.970286671637149212, 22.89273732682886475 ) ) ;
#3492=CARTESIAN_POINT ( 'NONE',  ( 9.999999999999998224, -6.666666666666693608, 23.00000000000000000 ) ) ;
#3493=EDGE_CURVE ( 'NONE', #2868, #5932, #1189, .T. ) ;
#3497=CARTESIAN_POINT ( 'NONE',  ( -11.85339260696609287, 0.9193131588476503024, 30.72304697887226510 ) ) ;
#3501=CARTESIAN_POINT ( 'NONE',  ( 8.963431230391419646, 4.154428044945160714, 23.04275563843252783 ) ) ;
#3506=CARTESIAN_POINT ( 'NONE',  ( -2.035630462091350790, -14.63234267792704735, 38.34842398122203377 ) ) ;
#3510=CARTESIAN_POINT ( 'NONE',  ( 11.94400843721214756, 8.542271628752923007, 38.10037361971538417 ) ) ;
#3517=EDGE_LOOP ( 'NONE', ( #1555, #3293, #4891, #5714, #2485 ) ) ;
#3519=CARTESIAN_POINT ( 'NONE',  ( 9.930636381741159369, -5.809855716632679190, 22.73823205004162418 ) ) ;
#3520=DIRECTION ( 'NONE',  ( 0.000000000000000000, 0.000000000000000000, 1.000000000000000000 ) ) ;
#3525=CARTESIAN_POINT ( 'NONE',  ( -13.77854189090673742, 6.848566431882100464E-15, 35.81030296219172726 ) ) ;
#3528=CARTESIAN_POINT ( 'NONE',  ( -9.086808451283777899, 11.58129469348872753, 38.17632780249462598 ) ) ;
#3534=CARTESIAN_POINT ( 'NONE',  ( 10.16165675636470489, 6.925838250501023197, 28.06531976343183743 ) ) ;
#3541=CARTESIAN_POINT ( 'NONE',  ( -1.776706711792240379, -10.85317354580219451, 28.17414650202874782 ) ) ;
#3548=SHAPE_DEFINITION_REPRESENTATION ( #3191, #5596 ) ;
#3553=ORIENTED_EDGE ( 'NONE', *, *, #3189, .T. ) ;
#3555=CARTESIAN_POINT ( 'NONE',  ( 9.930636381741159369, 5.809855716632613465, 22.73823205004162418 ) ) ;
#3557=ORIENTED_EDGE ( 'NONE', *, *, #1371, .F. ) ;
#3559=CARTESIAN_POINT ( 'NONE',  ( -11.69030472852370828, 2.742560498089769538, 30.70728637550628548 ) ) ;
#3564=CARTESIAN_POINT ( 'NONE',  ( 9.554965159330777169, 6.787634061845148281, 25.51646427192168431 ) ) ;
#3567=CARTESIAN_POINT ( 'NONE',  ( -9.144590365090015993, 9.969668718019493170, 22.73823205004162418 ) ) ;
#3568=EDGE_CURVE ( 'NONE', #5932, #5813, #1215, .T. ) ;
#3569=CARTESIAN_POINT ( 'NONE',  ( 2.035738251814313671, -14.63232105816060979, 38.34842656511671066 ) ) ;
#3581=EDGE_LOOP ( 'NONE', ( #2867, #984, #1108, #4264 ) ) ;
#3582=CARTESIAN_POINT ( 'NONE',  ( 9.515772848102855619, 10.27564057804868902, 33.05475024408053031 ) ) ;
#3585=ORIENTED_EDGE ( 'NONE', *, *, #1398, .T. ) ;
#3587=CARTESIAN_POINT ( 'NONE',  ( -8.967351122863068014, 7.487361748921663285, 22.92808036848186504 ) ) ;
#3594=EDGE_LOOP ( 'NONE', ( #2918, #3925, #306, #696 ) ) ;
#3597=CARTESIAN_POINT ( 'NONE',  ( 0.000000000000000000, 0.000000000000000000, 205.0000000000000568 ) ) ;
#3601=DIRECTION ( 'NONE',  ( -0.000000000000000000, -1.000000000000000000, -0.000000000000000000 ) ) ;
#3607=EDGE_CURVE ( 'NONE', #882, #1611, #3432, .T. ) ;
#3610=FACE_OUTER_BOUND ( 'NONE', #4983, .T. ) ;
#3612=CARTESIAN_POINT ( 'NONE',  ( 14.42236408824967597, -3.019346778933470254, 38.33740271606987449 ) ) ;
#3613=CARTESIAN_POINT ( 'NONE',  ( -9.554964866038103466, 6.787591074359464294, 25.51646829178083564 ) ) ;
#3623=CARTESIAN_POINT ( 'NONE',  ( -9.166666666666657193, 9.999999999999998224, 23.00000000000000000 ) ) ;
#3626=CARTESIAN_POINT ( 'NONE',  ( -7.570044180282074819, -12.64059746256323002, 38.23931193745811186 ) ) ;
#3639=CARTESIAN_POINT ( 'NONE',  ( -9.999999999999998224, -9.999999999999998224, 23.00000000000000000 ) ) ;
#3640=ORIENTED_EDGE ( 'NONE', *, *, #1901, .F. ) ;
#3644=CARTESIAN_POINT ( 'NONE',  ( 9.928243323025455425, 0.8581648076837078420, 25.63579099555274965 ) ) ;
#3645=EDGE_CURVE ( 'NONE', #4944, #3749, #3397, .T. ) ;
#3647=CARTESIAN_POINT ( 'NONE',  ( -11.57174281757876955, 8.159736356077658570, 35.66679457777021867 ) ) ;
#3649=CARTESIAN_POINT ( 'NONE',  ( -7.228764404800519294, 11.39256393965315439, 33.15620429642044797 ) ) ;
#3673=CARTESIAN_POINT ( 'NONE',  ( 10.70751178813581284, -3.531766105781286136, 28.15279191876807374 ) ) ;
#3674=CARTESIAN_POINT ( 'NONE',  ( -11.39263409468386712, 7.228600378928585535, 33.15620577507544908 ) ) ;
#3676=CARTESIAN_POINT ( 'NONE',  ( -7.570233152424900247, 12.64046943599296924, 38.23931941266579315 ) ) ;
#3680=DIRECTION ( 'NONE',  ( -0.000000000000000000, -0.000000000000000000, -1.000000000000000000 ) ) ;
#3682=CARTESIAN_POINT ( 'NONE',  ( -13.92731518891510945, 4.729006349282765420, 38.16144984630088288 ) ) ;
#3684=UNCERTAINTY_MEASURE_WITH_UNIT (LENGTH_MEASURE( 1.000000000000000082E-05 ), #1802, 'distance_accuracy_value', 'NONE');
#3685=CARTESIAN_POINT ( 'NONE',  ( -6.400535080091638740, -11.71455171164206810, 33.18278799730942552 ) ) ;
#3690=CYLINDRICAL_SURFACE ( 'NONE', #2163, 15.67638808697555142 ) ;
#3692=DIRECTION ( 'NONE',  ( -0.000000000000000000, -0.000000000000000000, -1.000000000000000000 ) ) ;
#3693=CARTESIAN_POINT ( 'NONE',  ( -9.999999999999998224, 8.333333333333346360, 23.00000000000000000 ) ) ;
#3695=ORIENTED_EDGE ( 'NONE', *, *, #675, .F. ) ;
#3698=CARTESIAN_POINT ( 'NONE',  ( 7.765009959110445337, 12.46305503907310452, 38.11687012676380704 ) ) ;
#3699=CARTESIAN_POINT ( 'NONE',  ( 12.24723121994938779, -4.666652649023727228, 33.22501677959694177 ) ) ;
#3702=CARTESIAN_POINT ( 'NONE',  ( -5.533593864557652786, 11.98089146579573061, 33.20390238845318720 ) ) ;
#3708=CARTESIAN_POINT ( 'NONE',  ( -13.16326790094652210, 6.508032323544350461, 38.13839276770976028 ) ) ;
#3711=CARTESIAN_POINT ( 'NONE',  ( -7.077172123266715964, -10.77715421822219710, 30.61076540981939687 ) ) ;
#3712=ORIENTED_EDGE ( 'NONE', *, *, #5637, .F. ) ;
#3727=CARTESIAN_POINT ( 'NONE',  ( 9.999999999999998224, -9.999999999999998224, -167.0000000000000284 ) ) ;
#3732=CARTESIAN_POINT ( 'NONE',  ( 11.98089146579572883, -5.533593864557682096, 33.20390238845318009 ) ) ;
#3733=CARTESIAN_POINT ( 'NONE',  ( -8.983694681928700021, 9.994658916190592990, 22.80938439471025703 ) ) ;
#3745=CARTESIAN_POINT ( 'NONE',  ( 10.27564057804868725, 9.515772848102850290, 33.05475024408053741 ) ) ;
#3749=VERTEX_POINT ( 'NONE', #5807 ) ;
#3753=( NAMED_UNIT ( * ) PLANE_ANGLE_UNIT ( ) SI_UNIT ( $, .RADIAN. ) );
#3763=DIRECTION ( 'NONE',  ( 0.000000000000000000, 0.000000000000000000, 1.000000000000000000 ) ) ;
#3768=CARTESIAN_POINT ( 'NONE',  ( -6.652779355836718977, 8.964415603276487232, 22.96342386064221941 ) ) ;
#3773=CARTESIAN_POINT ( 'NONE',  ( -11.12736491637287983, -8.926329112024045997, 35.63514765224429226 ) ) ;
#3774=CARTESIAN_POINT ( 'NONE',  ( -10.37777353962637505, 10.37777353962536608, 38.05103295300745003 ) ) ;
#3777=CARTESIAN_POINT ( 'NONE',  ( 6.488003555186288906, -13.19914683770228336, 38.13881399654477633 ) ) ;
#3784=CARTESIAN_POINT ( 'NONE',  ( 4.399300199984971016, -10.59948853791303769, 28.13666499103235452 ) ) ;
#3785=ADVANCED_FACE ( 'NONE', ( #3428 ), #1087, .T. ) ;
#3786=EDGE_CURVE ( 'NONE', #6095, #4944, #901, .T. ) ;
#3792=CARTESIAN_POINT ( 'NONE',  ( 10.19629538396769952, 10.19629538384312184, 35.54424335298406135 ) ) ;
#3793=CARTESIAN_POINT ( 'NONE',  ( 12.01622299351614132, -7.392961014695930366, 35.69843844696170976 ) ) ;
#3794=EDGE_CURVE ( 'NONE', #251, #4467, #5216, .T. ) ;
#3795=EDGE_CURVE ( 'NONE', #1157, #936, #615, .T. ) ;
#3796=ORIENTED_EDGE ( 'NONE', *, *, #1680, .F. ) ;
#3797=CARTESIAN_POINT ( 'NONE',  ( 4.154433491267528034, 8.963431154120575783, 23.04275521548131067 ) ) ;
#3798=CARTESIAN_POINT ( 'NONE',  ( -2.164213882025733060, 15.56315586465741951, 38.00000000000000711 ) ) ;
#3799=CARTESIAN_POINT ( 'NONE',  ( -13.90645689909058369, -4.715863500832077726, 38.16097513848706058 ) ) ;
#3803=CARTESIAN_POINT ( 'NONE',  ( -10.50531938289192446, -7.869812776064875948, 30.57803900350706172 ) ) ;
#3806=CARTESIAN_POINT ( 'NONE',  ( 9.999999999999998224, -9.999999999999998224, 23.00000000000000000 ) ) ;
#3807=CARTESIAN_POINT ( 'NONE',  ( 1.900794651634724719, -14.58443831393950418, 38.18056006088391996 ) ) ;
#3816=CARTESIAN_POINT ( 'NONE',  ( 10.38144361273100280, -10.38144361273100813, 38.10175261887127363 ) ) ;
#3821=PLANE ( 'NONE',  #1472 ) ;
#3827=CARTESIAN_POINT ( 'NONE',  ( 9.554964866038103466, -6.787591074359449195, 25.51646829178083564 ) ) ;
#3831=CARTESIAN_POINT ( 'NONE',  ( -0.8880320553140206297, 10.89081796499577415, 28.17941898721253580 ) ) ;
#3838=CARTESIAN_POINT ( 'NONE',  ( -10.16165675636470134, -6.925838250501020532, 28.06531976343184098 ) ) ;
#3839=CARTESIAN_POINT ( 'NONE',  ( 8.069545871843425644, -13.47611570251764412, 37.99999999999999289 ) ) ;
#3843=AXIS2_PLACEMENT_3D ( 'NONE', #4097, #5109, #6013 ) ;
#3846=LINE ( 'NONE', #5796, #4346 ) ;
#3847=VECTOR ( 'NONE', #1071, 1000.000000000000000 ) ;
#3853=CARTESIAN_POINT ( 'NONE',  ( 8.662324224478984647, -10.23352841777491840, 30.54531597708798429 ) ) ;
#3858=CARTESIAN_POINT ( 'NONE',  ( -9.999999999999998224, -8.999999999999998224, 23.00000000000000000 ) ) ;
#3860=CARTESIAN_POINT ( 'NONE',  ( -10.37777353962477278, -10.37777353962696303, 38.05103295300743582 ) ) ;
#3864=CARTESIAN_POINT ( 'NONE',  ( 11.03292118881348394, -8.007183658747754507, 33.12420745160152791 ) ) ;
#3866=CARTESIAN_POINT ( 'NONE',  ( 2.654236408786762702, 10.78034266696900367, 28.16346921039841078 ) ) ;
#3882=CARTESIAN_POINT ( 'NONE',  ( 9.000000000000005329, -8.999999999988066435, 23.06137295785747554 ) ) ;
#3884=CARTESIAN_POINT ( 'NONE',  ( 8.321944142006520551, -8.970286642449650572, 22.89273687632151422 ) ) ;
#3887=ORIENTED_EDGE ( 'NONE', *, *, #5176, .F. ) ;
#3892=CARTESIAN_POINT ( 'NONE',  ( 11.58116666691846319, -9.086997423426607767, 38.17633527770230017 ) ) ;
#3895=CARTESIAN_POINT ( 'NONE',  ( 5.845970755595366164, 13.50805179034378867, 38.28811402100272687 ) ) ;
#3896=CARTESIAN_POINT ( 'NONE',  ( 9.999999999999998224, 9.166666666666657193, 23.00000000000000000 ) ) ;
#3900=CARTESIAN_POINT ( 'NONE',  ( -13.07368784376654780, -4.807938790076510926, 35.76776929191790089 ) ) ;
#3902=CARTESIAN_POINT ( 'NONE',  ( 4.166666666666626107, -9.999999999999998224, 23.00000000000000000 ) ) ;
#3904=CARTESIAN_POINT ( 'NONE',  ( 13.33506331686138147, 3.878911688431560201, 35.78373290693656372 ) ) ;
#3905=CARTESIAN_POINT ( 'NONE',  ( 8.999999999999998224, -8.999999999999998224, 23.00000000000000000 ) ) ;
#3912=CARTESIAN_POINT ( 'NONE',  ( 9.086808451283770793, -11.58129469348872220, 38.17632780249461888 ) ) ;
#3914=CARTESIAN_POINT ( 'NONE',  ( -9.378998278013591872, 10.08321815271041721, 27.91486726096250948 ) ) ;
#3925=ORIENTED_EDGE ( 'NONE', *, *, #5261, .T. ) ;
#3926=CARTESIAN_POINT ( 'NONE',  ( 2.830884587392778595, 12.60026679007841643, 33.25110354061416018 ) ) ;
#3928=CARTESIAN_POINT ( 'NONE',  ( -12.74784844745956747, -7.336363311097503725, 38.12594328983445280 ) ) ;
#3934=CARTESIAN_POINT ( 'NONE',  ( -9.908812100099982700, -1.716690548177160824, 25.63028262842344773 ) ) ;
#3937=CARTESIAN_POINT ( 'NONE',  ( -5.273949241992683667, -14.79903580929011930, 38.00000000000000711 ) ) ;
#3940=CARTESIAN_POINT ( 'NONE',  ( 10.59948853791303769, 4.399300199984972792, 28.13666499103235452 ) ) ;
#3946=CARTESIAN_POINT ( 'NONE',  ( -5.842721101324136525E-14, -9.928243323025430556, 25.63579099555279583 ) ) ;
#3949=ORIENTED_EDGE ( 'NONE', *, *, #3473, .F. ) ;
#3954=AXIS2_PLACEMENT_3D ( 'NONE', #2206, #978, #1886 ) ;
#3955=DIRECTION ( 'NONE',  ( 0.000000000000000000, 0.000000000000000000, 1.000000000000000000 ) ) ;
#3956=DIRECTION ( 'NONE',  ( 0.000000000000000000, 0.000000000000000000, 1.000000000000000000 ) ) ;
#3957=VECTOR ( 'NONE', #576, 1000.000000000000000 ) ;
#3959=VECTOR ( 'NONE', #920, 1000.000000000000000 ) ;
#3968=CARTESIAN_POINT ( 'NONE',  ( -11.69030472852370295, -2.742560498089724241, 30.70728637550628193 ) ) ;
#3971=CARTESIAN_POINT ( 'NONE',  ( -4.147343260682193389, -9.916251082295019614, 22.73823205004162773 ) ) ;
#3972=CARTESIAN_POINT ( 'NONE',  ( 11.57174281757876955, 8.159736356077653241, 35.66679457777021867 ) ) ;
#3976=CARTESIAN_POINT ( 'NONE',  ( -1.716658579843648003, -9.908812303639328078, 25.63028407385523266 ) ) ;
#3984=DIRECTION ( 'NONE',  ( 1.000000000000000000, 0.000000000000000000, 0.000000000000000000 ) ) ;
#3990=CARTESIAN_POINT ( 'NONE',  ( 9.999999999999998224, 6.666666666666638541, 23.00000000000000000 ) ) ;
#3991=DIRECTION ( 'NONE',  ( 0.000000000000000000, 0.000000000000000000, 1.000000000000000000 ) ) ;
#3995=CARTESIAN_POINT ( 'NONE',  ( -12.74240908541723805, -1.902479615894477893, 33.26151609189631841 ) ) ;
#3998=EDGE_CURVE ( 'NONE', #2972, #5395, #3178, .T. ) ;
#3999=CARTESIAN_POINT ( 'NONE',  ( 9.462636878983097688, 7.610208295502463471, 25.48187184588751464 ) ) ;
#4003=CARTESIAN_POINT ( 'NONE',  ( -3.531766105781287468, -10.70751178813581461, 28.15279191876807729 ) ) ;
#4011=CARTESIAN_POINT ( 'NONE',  ( 9.000000000000005329, -8.999999999988066435, 23.06137295785747554 ) ) ;
#4019=CARTESIAN_POINT ( 'NONE',  ( -14.21240711833873505, -4.002955306052623285, 38.32637886702301699 ) ) ;
#4027=CARTESIAN_POINT ( 'NONE',  ( 8.963498645742985715, 4.986905650496026965, 23.01829711214647745 ) ) ;
#4032=EDGE_CURVE ( 'NONE', #1950, #936, #4605, .T. ) ;
#4034=CARTESIAN_POINT ( 'NONE',  ( -0.9505942623812230208, -12.81596724893641515, 33.26667497053199440 ) ) ;
#4045=CARTESIAN_POINT ( 'NONE',  ( 9.419333092093010507, 9.933255351449998827, 30.50691708577705796 ) ) ;
#4053=CARTESIAN_POINT ( 'NONE',  ( -10.46302782743270754, 5.247549479766074221, 28.11481907968152782 ) ) ;
#4056=CARTESIAN_POINT ( 'NONE',  ( -10.13908112636437053, 9.618700053625529378, 30.46372964425718521 ) ) ;
#4064=CARTESIAN_POINT ( 'NONE',  ( -9.696021465980070531, 12.35760627049922533, 37.99999999999999289 ) ) ;
#4066=CARTESIAN_POINT ( 'NONE',  ( -1.955660088736181144E-14, -12.81596724893641515, 33.26667497053200151 ) ) ;
#4068=CARTESIAN_POINT ( 'NONE',  ( -9.000000000000005329, 8.999999999988014920, 23.06137295785748265 ) ) ;
#4071=DIRECTION ( 'NONE',  ( 1.000000000000000000, 0.000000000000000000, 0.000000000000000000 ) ) ;
#4073=CARTESIAN_POINT ( 'NONE',  ( -14.79903580929012463, 5.273949241992682779, 38.00000000000001421 ) ) ;
#4077=CARTESIAN_POINT ( 'NONE',  ( 9.999999999999998224, -9.999999999999998224, 23.00000000000000000 ) ) ;
#4078=B_SPLINE_SURFACE_WITH_KNOTS ( 'NONE', 3, 3, ( 
 ( #539, #57, #1878, #1002, #2417, #1383, #467 ),
 ( #4754, #436, #5755, #4306, #3288, #5660, #5259 ),
 ( #5788, #3773, #5193, #966, #3405, #1416, #1907 ),
 ( #2353, #4243, #6140, #3803, #5718, #1446, #1942 ),
 ( #3348, #1032, #2883, #1481, #3838, #3377, #2911 ),
 ( #5290, #4816, #569, #2789, #250, #2122, #2488 ),
 ( #2067, #5386, #4890, #2515, #1538, #1126, #4914 ),
 ( #4946, #3900, #5411, #1147, #606, #4375, #4403 ),
 ( #4019, #1099, #2606, #125, #1177, #223, #725 ),
 ( #3006, #151, #663, #3968, #5942, #2033, #2980 ),
 ( #4470, #4496, #3995, #3443, #2543, #3934, #5884 ),
 ( #5853, #1063, #4437, #2096, #1600, #1572, #1657 ),
 ( #3474, #3525, #694, #3032, #4857, #192, #5909 ),
 ( #4978, #2576, #5353, #3497, #1622, #5815, #5443 ),
 ( #3069, #638, #5317, #2945, #2005, #402, #2279 ),
 ( #6083, #4171, #2248, #3559, #315, #5005, #3159 ),
 ( #4108, #1233, #3186, #1208, #4525, #4648, #1287 ),
 ( #2662, #2717, #867, #4146, #1687, #1261, #2193 ),
 ( #5095, #4615, #342, #6059, #4053, #2217, #841 ),
 ( #3124, #5972, #4560, #1780, #4084, #6028, #370 ),
 ( #5588, #1749, #3674, #1313, #3214, #3613, #5121 ),
 ( #2750, #3647, #815, #5067, #2691, #5478, #3587 ),
 ( #3098, #5505, #750, #2632, #281, #2158, #5036 ),
 ( #783, #5998, #1712, #5534, #4589, #5563, #1832 ),
 ( #4901, #5613, #4419, #2922, #3914, #5774, #3733 ) ),
 .UNSPECIFIED., .F., .F., .F.,
 ( 4, 3, 3, 3, 3, 3, 3, 3, 4 ),
 ( 4, 3, 4 ),
 ( 0.000000000000000000, 0.1250000000000000000, 0.2500000000000000000, 0.3750000000000000000, 0.5000000000000000000, 0.6250000000000000000, 0.7500000000000000000, 0.8750000000000000000, 1.000000000000000000 ),
 ( 0.000000000000000000, 0.5087255983319458608, 1.017451196663891722 ),
 .UNSPECIFIED. ) ;
#4079=CARTESIAN_POINT ( 'NONE',  ( -3.314202382262247060, 14.30535051437897742, 38.17196567842750454 ) ) ;
#4083=CARTESIAN_POINT ( 'NONE',  ( 8.963498645742985715, -4.986905650496099796, 23.01829711214647745 ) ) ;
#4084=CARTESIAN_POINT ( 'NONE',  ( -10.32655419438761690, 6.095889600840175504, 28.09296952102860345 ) ) ;
#4092=CARTESIAN_POINT ( 'NONE',  ( -9.515772848102853843, -10.27564057804868902, 33.05475024408053741 ) ) ;
#4097=CARTESIAN_POINT ( 'NONE',  ( 0.000000000000000000, 0.000000000000000000, 205.0000000000000568 ) ) ;
#4100=CARTESIAN_POINT ( 'NONE',  ( -15.67638808697554786, 1.082228759108216254, 38.00000000000000711 ) ) ;
#4107=CARTESIAN_POINT ( 'NONE',  ( 11.42336634021359032, -4.532931003857849639, 30.68084270896568810 ) ) ;
#4108=CARTESIAN_POINT ( 'NONE',  ( -14.21238549857230993, 4.003063095775585722, 38.32638145091770809 ) ) ;
#4109=ORIENTED_EDGE ( 'NONE', *, *, #181, .F. ) ;
#4110=CARTESIAN_POINT ( 'NONE',  ( -4.533051537554481314, 11.42333844578497626, 30.68084101284746623 ) ) ;
#4119=MANIFOLD_SOLID_BREP ( 'Shell1', #1755 ) ;
#4120=AXIS2_PLACEMENT_3D ( 'NONE', #2627, #3520, #5475 ) ;
#4125=PRODUCT ( 'tube', 'tube', '', ( #768 ) ) ;
#4128=ORIENTED_EDGE ( 'NONE', *, *, #2593, .F. ) ;
#4133=DIRECTION ( 'NONE',  ( -1.000000000000000000, 0.000000000000000000, 0.000000000000000000 ) ) ;
#4142=CARTESIAN_POINT ( 'NONE',  ( -9.676903716103852915, 11.04476983075539565, 38.07288907902119490 ) ) ;
#4143=CARTESIAN_POINT ( 'NONE',  ( 11.85339260696609465, -0.9193131588476518568, 30.72304697887226510 ) ) ;
#4146=CARTESIAN_POINT ( 'NONE',  ( -11.42336634021359387, 4.532931003857847863, 30.68084270896569521 ) ) ;
#4148=CARTESIAN_POINT ( 'NONE',  ( -2.654236408786703194, 10.78034266696900012, 28.16346921039841078 ) ) ;
#4151=CIRCLE ( 'NONE', #1181, 14.67638808697554964 ) ;
#4156=CARTESIAN_POINT ( 'NONE',  ( -8.432825516645550579, -9.370308891928099015, 25.44727539999420074 ) ) ;
#4159=ORIENTED_EDGE ( 'NONE', *, *, #6093, .T. ) ;
#4163=CARTESIAN_POINT ( 'NONE',  ( -9.999999999999998224, -0.8333333333332838544, 23.00000000000000000 ) ) ;
#4170=CARTESIAN_POINT ( 'NONE',  ( 9.928243323025451872, -0.8581648076837659067, 25.63579099555280649 ) ) ;
#4171=CARTESIAN_POINT ( 'NONE',  ( -13.51119013911331024, 2.923529524533194923, 35.79437308157104525 ) ) ;
#4173=CARTESIAN_POINT ( 'NONE',  ( -1.839621235173124703, 11.79778917763282209, 30.71783072571432882 ) ) ;
#4180=EDGE_CURVE ( 'NONE', #5932, #3300, #3296, .T. ) ;
#4181=CARTESIAN_POINT ( 'NONE',  ( -9.245260337044127752, -9.269614772507658529, 25.40693856330804934 ) ) ;
#4183=DIRECTION ( 'NONE',  ( 0.000000000000000000, 1.000000000000000000, 0.000000000000000000 ) ) ;
#4189=CARTESIAN_POINT ( 'NONE',  ( -9.916251082295017838, -4.147343260682107235, 22.73823205004162418 ) ) ;
#4194=CARTESIAN_POINT ( 'NONE',  ( 4.735139425640385369, 13.92517021172140446, 38.16137691020119860 ) ) ;
#4195=CARTESIAN_POINT ( 'NONE',  ( 13.51119013911330846, -2.923529524533198476, 35.79437308157105235 ) ) ;
#4199=CARTESIAN_POINT ( 'NONE',  ( -4.986905650496027853, 8.963498645742985715, 23.01829711214647745 ) ) ;
#4221=PLANE ( 'NONE',  #2873 ) ;
#4224=VECTOR ( 'NONE', #1294, 1000.000000000000000 ) ;
#4235=CARTESIAN_POINT ( 'NONE',  ( -4.954970571217796937, 13.90079966151758128, 38.30990426830500439 ) ) ;
#4236=B_SPLINE_CURVE_WITH_KNOTS ( 'NONE', 3,
 ( #671, #133, #5917, #1632, #5454, #1186 ),
 .UNSPECIFIED., .F., .F.,
 ( 4, 2, 4 ),
 ( 0.002357188415687188742, 0.01135824717474478128, 0.02035930593380237338 ),
 .UNSPECIFIED. ) ;
#4241=DIRECTION ( 'NONE',  ( -1.000000000000000000, 0.000000000000000000, 0.000000000000000000 ) ) ;
#4243=CARTESIAN_POINT ( 'NONE',  ( -11.57174281757876599, -8.159736356077647912, 35.66679457777020446 ) ) ;
#4246=UNCERTAINTY_MEASURE_WITH_UNIT (LENGTH_MEASURE( 1.000000000000000082E-05 ), #1819, 'distance_accuracy_value', 'NONE');
#4254=DIRECTION ( 'NONE',  ( 0.000000000000000000, 0.000000000000000000, 1.000000000000000000 ) ) ;
#4257=CARTESIAN_POINT ( 'NONE',  ( -8.999999999999998224, 0.000000000000000000, -167.0000000000000284 ) ) ;
#4261=CARTESIAN_POINT ( 'NONE',  ( 14.55721289103181348, -1.928061058260302607, 38.18004976450265531 ) ) ;
#4263=CARTESIAN_POINT ( 'NONE',  ( 4.533051537554480426, -11.42333844578497448, 30.68084101284746978 ) ) ;
#4264=ORIENTED_EDGE ( 'NONE', *, *, #2517, .F. ) ;
#4266=DIRECTION ( 'NONE',  ( 0.000000000000000000, -0.000000000000000000, 1.000000000000000000 ) ) ;
#4273=CARTESIAN_POINT ( 'NONE',  ( 4.954793796408216267, 13.90087379555094849, 38.30989703917857270 ) ) ;
#4275=CARTESIAN_POINT ( 'NONE',  ( 6.666666666666693608, 9.999999999999998224, 23.00000000000000000 ) ) ;
#4281=CARTESIAN_POINT ( 'NONE',  ( 9.269614772507654976, 9.245260337044125976, 25.40693856330804223 ) ) ;
#4286=DIRECTION ( 'NONE',  ( -0.000000000000000000, -0.000000000000000000, -1.000000000000000000 ) ) ;
#4290=CARTESIAN_POINT ( 'NONE',  ( 7.869812776064875948, -10.50531938289192624, 30.57803900350706527 ) ) ;
#4298=CARTESIAN_POINT ( 'NONE',  ( 10.12138240269938549, -10.27356722921338950, 35.55812462721154787 ) ) ;
#4301=CARTESIAN_POINT ( 'NONE',  ( 3.879012780925822579, 13.33504572891042272, 35.78373437249953781 ) ) ;
#4302=CARTESIAN_POINT ( 'NONE',  ( 9.166666666666673180, 9.999999999999998224, 23.00000000000000000 ) ) ;
#4304=EDGE_LOOP ( 'NONE', ( #4556, #1421, #4735, #692, #1967 ) ) ;
#4306=CARTESIAN_POINT ( 'NONE',  ( -9.933255351449995274, -9.419333092093001625, 30.50691708577705086 ) ) ;
#4310=CARTESIAN_POINT ( 'NONE',  ( 10.38144361273100635, 10.38144361273100635, 38.10175261887127363 ) ) ;
#4311=CARTESIAN_POINT ( 'NONE',  ( -7.356224370873720275, -12.70872189800991059, 38.12480727770462607 ) ) ;
#4317=ORIENTED_EDGE ( 'NONE', *, *, #1979, .F. ) ;
#4319=CARTESIAN_POINT ( 'NONE',  ( 3.322926169935022322, -8.964120776013638547, 23.06129021161081383 ) ) ;
#4321=EDGE_LOOP ( 'NONE', ( #3253, #5752, #4930, #2264, #5951, #384 ) ) ;
#4330=CARTESIAN_POINT ( 'NONE',  ( 12.11088206474084394, -8.328520801854338629, 38.20782360758020246 ) ) ;
#4331=EDGE_CURVE ( 'NONE', #3160, #1611, #2314, .T. ) ;
#4335=CARTESIAN_POINT ( 'NONE',  ( 0.9833031778629314212, 13.77854189090673742, 35.81030296219172726 ) ) ;
#4336=CARTESIAN_POINT ( 'NONE',  ( -4.260267006495014996, 15.12434353048566571, 38.00000000000000711 ) ) ;
#4343=CARTESIAN_POINT ( 'NONE',  ( 5.809855716632613465, -9.930636381741159369, 22.73823205004162773 ) ) ;
#4346=VECTOR ( 'NONE', #3295, 1000.000000000000000 ) ;
#4347=CARTESIAN_POINT ( 'NONE',  ( 10.03503361918882320, -10.72051346006293571, 38.06197354439399305 ) ) ;
#4356=CARTESIAN_POINT ( 'NONE',  ( 7.732441893382014264, -9.977717576970368540, 28.03187055541259909 ) ) ;
#4366=CARTESIAN_POINT ( 'NONE',  ( 8.975362584346067152, -9.157688896001753065, 22.85246612729342885 ) ) ;
#4367=ORIENTED_EDGE ( 'NONE', *, *, #248, .F. ) ;
#4369=CARTESIAN_POINT ( 'NONE',  ( -1.660911000355770772, 8.965240827029074211, 23.08598180255751942 ) ) ;
#4370=CARTESIAN_POINT ( 'NONE',  ( 9.981067540164714202, 9.981067540164714202, 22.73823205004162418 ) ) ;
#4371=CARTESIAN_POINT ( 'NONE',  ( -14.58318388806637778, -1.909955344851256065, 38.18050947768618641 ) ) ;
#4375=CARTESIAN_POINT ( 'NONE',  ( -9.778265433844637755, -4.273103006804783277, 25.59105575288735324 ) ) ;
#4376=EDGE_LOOP ( 'NONE', ( #6043, #3208, #1522, #1171, #2858 ) ) ;
#4378=ADVANCED_FACE ( 'NONE', ( #2787 ), #6090, .T. ) ;
#4379=CARTESIAN_POINT ( 'NONE',  ( 14.21240711833874037, 4.002955306052626838, 38.32637886702303121 ) ) ;
#4386=VERTEX_POINT ( 'NONE', #4684 ) ;
#4388=CARTESIAN_POINT ( 'NONE',  ( 5.113933401365476250, -9.708537589994012507, 25.56820946177495912 ) ) ;
#4389=ORIENTED_EDGE ( 'NONE', *, *, #1901, .T. ) ;
#4398=CARTESIAN_POINT ( 'NONE',  ( 1.589281154371899412E-14, 12.81596724893641515, 33.26667497053200151 ) ) ;
#4399=CARTESIAN_POINT ( 'NONE',  ( -4.166666666666626107, 9.999999999999998224, 23.00000000000000000 ) ) ;
#4403=CARTESIAN_POINT ( 'NONE',  ( -8.963431230391419646, -4.154428044945158938, 23.04275563843252783 ) ) ;
#4406=CARTESIAN_POINT ( 'NONE',  ( 2.164213882025729951, -15.56315586465741951, 38.00000000000000711 ) ) ;
#4409=CARTESIAN_POINT ( 'NONE',  ( 10.32656711695237739, 6.095798759547078838, 28.09297316833070113 ) ) ;
#4417=CARTESIAN_POINT ( 'NONE',  ( 1.839621235173124036, -11.79778917763282386, 30.71783072571433237 ) ) ;
#4419=CARTESIAN_POINT ( 'NONE',  ( -9.858401829237468661, 10.19494410001831142, 33.01259202755186095 ) ) ;
#4430=CARTESIAN_POINT ( 'NONE',  ( 7.869812776064898152, 10.50531938289192802, 30.57803900350706527 ) ) ;
#4431=CARTESIAN_POINT ( 'NONE',  ( 10.00000000000000000, 0.8333333333332849646, 23.00000000000000355 ) ) ;
#4437=CARTESIAN_POINT ( 'NONE',  ( -12.81596724893641337, -0.9505942623811892700, 33.26667497053200151 ) ) ;
#4439=CARTESIAN_POINT ( 'NONE',  ( -4.260267006495018549, -15.12434353048566571, 38.00000000000000711 ) ) ;
#4441=CARTESIAN_POINT ( 'NONE',  ( 10.85316926984840791, 1.776762854451773510, 28.17414535953233923 ) ) ;
#4449=CARTESIAN_POINT ( 'NONE',  ( -3.577867169202164632E-15, -14.74111653287705792, 38.35393095385146012 ) ) ;
#4458=DIRECTION ( 'NONE',  ( 1.000000000000000000, 0.000000000000000000, 0.000000000000000000 ) ) ;
#4464=CARTESIAN_POINT ( 'NONE',  ( 11.73806315776973541, -10.43169748385511042, 38.00000000000000711 ) ) ;
#4467=VERTEX_POINT ( 'NONE', #3314 ) ;
#4470=CARTESIAN_POINT ( 'NONE',  ( -14.63232105816060802, -2.035738251814319000, 38.34842656511671066 ) ) ;
#4473=CARTESIAN_POINT ( 'NONE',  ( 13.07368784376655135, 4.807938790076512703, 35.76776929191790089 ) ) ;
#4478=CARTESIAN_POINT ( 'NONE',  ( -2.742560498089771315, -11.69030472852371005, 30.70728637550628903 ) ) ;
#4479=ORIENTED_EDGE ( 'NONE', *, *, #3998, .F. ) ;
#4490=CARTESIAN_POINT ( 'NONE',  ( 7.228600378928579318, 11.39263409468387245, 33.15620577507543487 ) ) ;
#4491=CARTESIAN_POINT ( 'NONE',  ( 9.900940235153615987, -0.8289898103094419657, 22.73823205004162418 ) ) ;
#4496=CARTESIAN_POINT ( 'NONE',  ( -13.68731696136523368, -1.968147360634810106, 35.80501325620552677 ) ) ;
#4498=CARTESIAN_POINT ( 'NONE',  ( -9.632247231687287581, 10.63625351335941893, 35.59852902770369099 ) ) ;
#4500=CARTESIAN_POINT ( 'NONE',  ( 11.98089146579572706, 5.533593864557656339, 33.20390238845318720 ) ) ;
#4504=CARTESIAN_POINT ( 'NONE',  ( -5.845970755595367052, -13.50805179034378511, 38.28811402100272687 ) ) ;
#4508=LINE ( 'NONE', #2021, #891 ) ;
#4516=CARTESIAN_POINT ( 'NONE',  ( 8.007183658747752730, 11.03292118881348749, 33.12420745160152791 ) ) ;
#4517=CARTESIAN_POINT ( 'NONE',  ( 9.999999999999998224, -1.666666666666713814, 23.00000000000000000 ) ) ;
#4525=CARTESIAN_POINT ( 'NONE',  ( -10.70751178813581284, 3.531766105781286580, 28.15279191876807374 ) ) ;
#4529=FACE_OUTER_BOUND ( 'NONE', #2386, .T. ) ;
#4533=PRODUCT_DEFINITION_FORMATION_WITH_SPECIFIED_SOURCE ( 'ANY', '', #4125, .NOT_KNOWN. ) ;
#4536=CARTESIAN_POINT ( 'NONE',  ( -5.833333333333301063, 9.999999999999998224, 23.00000000000000000 ) ) ;
#4539=CARTESIAN_POINT ( 'NONE',  ( 2.491918585145396214, -8.964680801521357267, 23.07363600708416840 ) ) ;
#4549=CARTESIAN_POINT ( 'NONE',  ( -9.999999999999998224, -6.666666666666634988, 23.00000000000000000 ) ) ;
#4553=CARTESIAN_POINT ( 'NONE',  ( 9.999999999999998224, 4.166666666666626107, 23.00000000000000000 ) ) ;
#4556=ORIENTED_EDGE ( 'NONE', *, *, #5458, .T. ) ;
#4557=CARTESIAN_POINT ( 'NONE',  ( 10.46302782743270576, -5.247549479766075109, 28.11481907968152427 ) ) ;
#4560=CARTESIAN_POINT ( 'NONE',  ( -11.71455171164206988, 6.400535080091636075, 33.18278799730943263 ) ) ;
#4563=CARTESIAN_POINT ( 'NONE',  ( -9.515772848102846737, 10.27564057804868725, 33.05475024408053741 ) ) ;
#4572=CARTESIAN_POINT ( 'NONE',  ( -8.007183658747754507, -11.03292118881348749, 33.12420745160152791 ) ) ;
#4575=CARTESIAN_POINT ( 'NONE',  ( 8.999999999999998224, 0.000000000000000000, -167.0000000000000284 ) ) ;
#4581=CARTESIAN_POINT ( 'NONE',  ( -9.900940235153615987, 0.8289898103094429649, 22.73823205004162418 ) ) ;
#4584=DIRECTION ( 'NONE',  ( 1.000000000000000000, 0.000000000000000000, 0.000000000000000000 ) ) ;
#4586=B_SPLINE_SURFACE_WITH_KNOTS ( 'NONE', 3, 1, ( 
 ( #1417, #1879, #5226 ),
 ( #1484, #1067, #1978 ),
 ( #1103, #2519, #129 ),
 ( #3839, #2007, #2982 ),
 ( #2912, #5758, #4343 ),
 ( #2451, #3902, #4892 ),
 ( #5388, #5818, #640 ),
 ( #4406, #3408, #4918 ),
 ( #665, #5319, #2070 ),
 ( #4859, #2546, #3378 ),
 ( #153, #5291, #2037 ),
 ( #4439, #2418, #194 ),
 ( #3937, #5855, #3971 ),
 ( #3476, #2947, #1033 ),
 ( #5886, #1003, #3349 ),
 ( #1128, #610, #4817 ),
 ( #3008, #572, #5262 ),
 ( #1576, #2490, #1542 ) ),
 .UNSPECIFIED., .F., .F., .F.,
 ( 4, 2, 2, 2, 2, 2, 2, 2, 4 ),
 ( 2, 1, 2 ),
 ( 0.000000000000000000, 0.1250000000000000000, 0.2500000000000000000, 0.3750000000000000000, 0.5000000000000000000, 0.6250000000000000000, 0.7500000000000000000, 0.8750000000000000000, 1.000000000000000000 ),
 ( 0.000000000000000000, 1.000000000000000000, 1.017451196663891499 ),
 .UNSPECIFIED. ) ;
#4588=CARTESIAN_POINT ( 'NONE',  ( 10.32655419438761690, -6.095889600840178169, 28.09296952102860701 ) ) ;
#4589=CARTESIAN_POINT ( 'NONE',  ( -9.590870124851306855, 9.322893336083163618, 27.95908392747358917 ) ) ;
#4591=CARTESIAN_POINT ( 'NONE',  ( -5.113933401365456710, 9.708537589994000072, 25.56820946177495557 ) ) ;
#4599=CARTESIAN_POINT ( 'NONE',  ( -10.38144361273100813, -10.38144361273100458, 38.10175261887127363 ) ) ;
#4605=LINE ( 'NONE', #303, #766 ) ;
#4613=CARTESIAN_POINT ( 'NONE',  ( 6.512188664277434924, 13.16119478149493993, 38.13833290264204834 ) ) ;
#4614=CARTESIAN_POINT ( 'NONE',  ( 8.965668681055127820, -5.138611361899592999E-14, 23.09216300389308785 ) ) ;
#4615=CARTESIAN_POINT ( 'NONE',  ( -12.74411457810409587, 5.685785403169732355, 35.74643938915853880 ) ) ;
#4617=CARTESIAN_POINT ( 'NONE',  ( -2.570253631893256951, 9.871311131128940985, 25.61911440830482789 ) ) ;
#4619=AXIS2_PLACEMENT_3D ( 'NONE', #5777, #5941, #1499 ) ;
#4630=CARTESIAN_POINT ( 'NONE',  ( -9.772747244158502156, -10.99573437649350183, 38.14042781937035187 ) ) ;
#4639=CARTESIAN_POINT ( 'NONE',  ( -9.910574073276151807, -3.317157231508557569, 22.73823205004162418 ) ) ;
#4642=DIRECTION ( 'NONE',  ( 0.000000000000000000, -0.000000000000000000, 1.000000000000000000 ) ) ;
#4646=CARTESIAN_POINT ( 'NONE',  ( 8.965668681055129596, 0.8304760625348918124, 23.09216300389309140 ) ) ;
#4648=CARTESIAN_POINT ( 'NONE',  ( -9.833809958618568103, 3.423848683943055971, 25.60794474275442667 ) ) ;
#4651=CARTESIAN_POINT ( 'NONE',  ( -7.393143600131252491, 12.01612071878465393, 35.69844150329612376 ) ) ;
#4662=CARTESIAN_POINT ( 'NONE',  ( -6.652784304366590185, -8.964415574088988592, 22.96342341013487243 ) ) ;
#4670=CARTESIAN_POINT ( 'NONE',  ( -9.958856949317492990, -8.309552794738944925, 22.73823205004162418 ) ) ;
#4676=CARTESIAN_POINT ( 'NONE',  ( 10.89081796499576882, 0.8880320553140124140, 28.17941898721253580 ) ) ;
#4680=CARTESIAN_POINT ( 'NONE',  ( -7.077301327650770801, 10.77711034800893053, 30.61076202992614270 ) ) ;
#4684=CARTESIAN_POINT ( 'NONE',  ( -14.67638808697555319, 1.484446970801598990E-11, 38.18288438803429585 ) ) ;
#4694=CARTESIAN_POINT ( 'NONE',  ( 0.000000000000000000, 0.000000000000000000, 205.0000000000000568 ) ) ;
#4702=CARTESIAN_POINT ( 'NONE',  ( 0.4914066504972167682, 14.67601930163248625, 38.18288424882400278 ) ) ;
#4704=CARTESIAN_POINT ( 'NONE',  ( -9.999999999999998224, 9.999999999999998224, 23.00000000000000000 ) ) ;
#4706=CARTESIAN_POINT ( 'NONE',  ( -3.645499761006327333, 11.58282027941459091, 30.69674202529824214 ) ) ;
#4707=CARTESIAN_POINT ( 'NONE',  ( -9.999999999999998224, 9.999999999999998224, 23.00000000000000000 ) ) ;
#4714=CARTESIAN_POINT ( 'NONE',  ( 14.67638808697554964, -1.485455082520059617E-11, 38.18288438803429585 ) ) ;
#4720=CARTESIAN_POINT ( 'NONE',  ( 8.975362584346067152, 9.157688896001733525, 22.85246612729342885 ) ) ;
#4723=VECTOR ( 'NONE', #1236, 1000.000000000000000 ) ;
#4733=CARTESIAN_POINT ( 'NONE',  ( 4.807938790076513591, -13.07368784376655491, 35.76776929191790089 ) ) ;
#4735=ORIENTED_EDGE ( 'NONE', *, *, #3794, .T. ) ;
#4744=CARTESIAN_POINT ( 'NONE',  ( 9.793760812180217101, -8.539139919159236314, 27.99841606626185353 ) ) ;
#4747=CARTESIAN_POINT ( 'NONE',  ( 5.070403286795210678E-14, 8.965668681055127820, 23.09216300389308785 ) ) ;
#4748=CARTESIAN_POINT ( 'NONE',  ( -4.147343260682110788, 9.916251082295017838, 22.73823205004162418 ) ) ;
#4754=CARTESIAN_POINT ( 'NONE',  ( -10.99573437649350005, -9.772747244158498603, 38.14042781937033766 ) ) ;
#4760=CARTESIAN_POINT ( 'NONE',  ( 9.000000000000005329, -8.999999999988066435, 23.06137295785747554 ) ) ;
#4761=CARTESIAN_POINT ( 'NONE',  ( 14.67638808697554964, 1.797339169375895343E-15, 205.0000000000000568 ) ) ;
#4765=DIRECTION ( 'NONE',  ( -0.07194996680737229811, 0.07194996680737240913, 0.9948097328398211037 ) ) ;
#4767=EDGE_LOOP ( 'NONE', ( #3712, #3227, #2344, #3796 ) ) ;
#4768=CARTESIAN_POINT ( 'NONE',  ( 14.67638808697554964, -1.485455082520059617E-11, 38.18288438803429585 ) ) ;
#4771=CARTESIAN_POINT ( 'NONE',  ( 6.248091806769201284, -11.02058084744346367, 30.63788045528724169 ) ) ;
#4772=ORIENTED_EDGE ( 'NONE', *, *, #3013, .F. ) ;
#4775=FACE_BOUND ( 'NONE', #910, .T. ) ;
#4778=CARTESIAN_POINT ( 'NONE',  ( 10.37777353962571425, 10.37777353962603044, 38.05103295300744293 ) ) ;
#4779=CARTESIAN_POINT ( 'NONE',  ( 10.23348454756165715, -8.662453428863083005, 30.54531259719474079 ) ) ;
#4781=CARTESIAN_POINT ( 'NONE',  ( 6.248212340465907566, 11.02055295301484428, 30.63787875916901626 ) ) ;
#4782=CARTESIAN_POINT ( 'NONE',  ( 0.8289898103094419657, 9.900940235153615987, 22.73823205004162418 ) ) ;
#4789=CARTESIAN_POINT ( 'NONE',  ( 7.333173243373136252, -12.74975250248365199, 38.12600698484704509 ) ) ;
#4792=DIRECTION ( 'NONE',  ( -1.000000000000000000, 0.000000000000000000, 0.000000000000000000 ) ) ;
#4797=CARTESIAN_POINT ( 'NONE',  ( 12.46477214039048853, -7.762281575598469985, 38.11692635423789710 ) ) ;
#4798=CARTESIAN_POINT ( 'NONE',  ( 9.419333092093003401, -9.933255351449997050, 30.50691708577705796 ) ) ;
#4810=CARTESIAN_POINT ( 'NONE',  ( -0.9505942623811894920, 12.81596724893641692, 33.26667497053200151 ) ) ;
#4811=CARTESIAN_POINT ( 'NONE',  ( 9.696021465980070531, 12.35760627049922178, 38.00000000000000000 ) ) ;
#4816=CARTESIAN_POINT ( 'NONE',  ( -12.41454131244164216, -6.563632016262936908, 35.72510948639917672 ) ) ;
#4817=CARTESIAN_POINT ( 'NONE',  ( -8.309552794738978676, -9.958856949317492990, 22.73823205004162773 ) ) ;
#4829=CARTESIAN_POINT ( 'NONE',  ( 9.772747244158500379, -10.99573437649350005, 38.14042781937034476 ) ) ;
#4832=ADVANCED_FACE ( 'NONE', ( #4529 ), #1298, .F. ) ;
#4842=CARTESIAN_POINT ( 'NONE',  ( 10.27564057804868725, -9.515772848102859172, 33.05475024408053031 ) ) ;
#4848=CARTESIAN_POINT ( 'NONE',  ( 1.660914622755446324, 8.965240787521256749, 23.08598164463087343 ) ) ;
#4849=CARTESIAN_POINT ( 'NONE',  ( 4.166666666666706931, 9.999999999999998224, 23.00000000000000000 ) ) ;
#4854=B_SPLINE_CURVE_WITH_KNOTS ( 'NONE', 3,
 ( #2908, #2483, #4371, #5255, #1904, #3799, #5713, #122, #3928, #1971, #1934, #2002, #1568, #1477 ),
 .UNSPECIFIED., .F., .F.,
 ( 4, 2, 2, 2, 2, 2, 4 ),
 ( 0.01144098757322556392, 0.01429571064770015186, 0.01572307218493744496, 0.01715043372217473980, 0.02000515679664932600, 0.02143251833388662084, 0.02285987987112391567 ),
 .UNSPECIFIED. ) ;
#4857=CARTESIAN_POINT ( 'NONE',  ( -10.89081796499577059, 3.137335681707220393E-14, 28.17941898721253580 ) ) ;
#4859=CARTESIAN_POINT ( 'NONE',  ( -1.082228759108218918, -15.67638808697554786, 38.00000000000000711 ) ) ;
#4861=FACE_OUTER_BOUND ( 'NONE', #224, .T. ) ;
#4862=CIRCLE ( 'NONE', #4955, 14.67638808697554964 ) ;
#4863=CARTESIAN_POINT ( 'NONE',  ( 10.37777353962609972, -10.37777353962564852, 38.05103295300747845 ) ) ;
#4869=CARTESIAN_POINT ( 'NONE',  ( 8.999999999999996447, -6.000548030722295145, 23.13502304888910643 ) ) ;
#4872=CARTESIAN_POINT ( 'NONE',  ( 5.390571672161841299, -11.22195964661421819, 30.65936073406735574 ) ) ;
#4880=DIRECTION ( 'NONE',  ( 1.000000000000000000, 0.000000000000000000, 0.000000000000000000 ) ) ;
#4882=ORIENTED_EDGE ( 'NONE', *, *, #3493, .T. ) ;
#4884=CARTESIAN_POINT ( 'NONE',  ( 4.986905650496099796, 8.963498645742985715, 23.01829711214647745 ) ) ;
#4885=CARTESIAN_POINT ( 'NONE',  ( 1.657983872361911803, 9.902916272933978803, 22.73823205004162418 ) ) ;
#4890=CARTESIAN_POINT ( 'NONE',  ( -11.98089146579572706, -5.533593864557662556, 33.20390238845318009 ) ) ;
#4891=ORIENTED_EDGE ( 'NONE', *, *, #895, .T. ) ;
#4892=CARTESIAN_POINT ( 'NONE',  ( 4.147343260682110788, -9.916251082295019614, 22.73823205004162773 ) ) ;
#4894=CARTESIAN_POINT ( 'NONE',  ( 11.42333844578497271, 4.533051537554481314, 30.68084101284746623 ) ) ;
#4899=CARTESIAN_POINT ( 'NONE',  ( -2.923529524533197588, -13.51119013911331024, 35.79437308157104525 ) ) ;
#4901=CARTESIAN_POINT ( 'NONE',  ( -10.38144361273100280, 10.38144361273100991, 38.10175261887127363 ) ) ;
#4903=CARTESIAN_POINT ( 'NONE',  ( 14.18603054855849699, 3.792815487221774973, 38.16899780669729836 ) ) ;
#4909=VERTEX_POINT ( 'NONE', #5903 ) ;
#4910=CARTESIAN_POINT ( 'NONE',  ( 10.08321815271041544, 9.378998278013591872, 27.91486726096250948 ) ) ;
#4911=CARTESIAN_POINT ( 'NONE',  ( 9.981067540164714202, -9.981067540164714202, 22.73823205004162418 ) ) ;
#4914=CARTESIAN_POINT ( 'NONE',  ( -8.963498645742985715, -4.986905650496026965, 23.01829711214648100 ) ) ;
#4918=CARTESIAN_POINT ( 'NONE',  ( 1.657983872361815880, -9.902916272933980579, 22.73823205004162773 ) ) ;
#4919=CARTESIAN_POINT ( 'NONE',  ( 13.68731696136523190, 1.968147360634808329, 35.80501325620552677 ) ) ;
#4925=CARTESIAN_POINT ( 'NONE',  ( -3.645573174172185738, -11.58281169573756131, 30.69674159737795804 ) ) ;
#4928=CARTESIAN_POINT ( 'NONE',  ( -10.37777353962637505, 10.37777353962536608, 38.05103295300745003 ) ) ;
#4929=VECTOR ( 'NONE', #1465, 1000.000000000000000 ) ;
#4930=ORIENTED_EDGE ( 'NONE', *, *, #3415, .F. ) ;
#4938=CARTESIAN_POINT ( 'NONE',  ( 7.392961014695930366, 12.01622299351614487, 35.69843844696170976 ) ) ;
#4940=CARTESIAN_POINT ( 'NONE',  ( 14.79903580929011930, -5.273949241992681891, 38.00000000000000711 ) ) ;
#4944=VERTEX_POINT ( 'NONE', #863 ) ;
#4946=CARTESIAN_POINT ( 'NONE',  ( -13.90079966151757596, -4.954970571217796937, 38.30990426830499729 ) ) ;
#4950=CARTESIAN_POINT ( 'NONE',  ( 10.50531938289192624, 7.869812776064879500, 30.57803900350706172 ) ) ;
#4955=AXIS2_PLACEMENT_3D ( 'NONE', #4694, #5297, #5730 ) ;
#4956=CARTESIAN_POINT ( 'NONE',  ( 0.9505942623811837189, -12.81596724893641515, 33.26667497053200151 ) ) ;
#4973=CARTESIAN_POINT ( 'NONE',  ( 9.999999999999998224, 5.833333333333301063, 23.00000000000000000 ) ) ;
#4978=CARTESIAN_POINT ( 'NONE',  ( -14.74111653287705792, 1.016991241531514323, 38.35393095385146012 ) ) ;
#4981=CARTESIAN_POINT ( 'NONE',  ( 8.964415603276487232, 6.652779355836718977, 22.96342386064221941 ) ) ;
#4983=EDGE_LOOP ( 'NONE', ( #4772, #4389, #5653, #3557 ) ) ;
#4986=CARTESIAN_POINT ( 'NONE',  ( 2.654236408786701862, -10.78034266696900190, 28.16346921039841433 ) ) ;
#4987=B_SPLINE_CURVE_WITH_KNOTS ( 'NONE', 3,
 ( #1524, #5871, #714, #207, #4903, #3424, #3019, #2531, #1641, #3510, #5896, #5337, #1114, #2592 ),
 .UNSPECIFIED., .F., .F.,
 ( 4, 2, 2, 2, 2, 2, 4 ),
 ( 0.01144098757322593515, 0.01429571064770019523, 0.01572307218493732700, 0.01715043372217445877, 0.02000515679664871885, 0.02143251833388584715, 0.02285987987112297892 ),
 .UNSPECIFIED. ) ;
#5000=CARTESIAN_POINT ( 'NONE',  ( 9.772747244158502156, 10.99573437649350183, 38.14042781937035187 ) ) ;
#5001=CARTESIAN_POINT ( 'NONE',  ( 9.958856949317492990, -8.309552794738978676, 22.73823205004162418 ) ) ;
#5005=CARTESIAN_POINT ( 'NONE',  ( -9.871311131128940985, 2.570253631893349322, 25.61911440830482789 ) ) ;
#5009=CARTESIAN_POINT ( 'NONE',  ( 11.02058084744346189, 6.248091806769200396, 30.63788045528724524 ) ) ;
#5014=CARTESIAN_POINT ( 'NONE',  ( -2.570253631893351098, -9.871311131128953420, 25.61911440830483144 ) ) ;
#5022=CARTESIAN_POINT ( 'NONE',  ( -11.73806315776973541, -10.43169748385510509, 37.99999999999999289 ) ) ;
#5023=ADVANCED_FACE ( 'NONE', ( #452 ), #6054, .F. ) ;
#5036=CARTESIAN_POINT ( 'NONE',  ( -8.970286671637149212, 8.321939193476739050, 22.89273732682886475 ) ) ;
#5039=CARTESIAN_POINT ( 'NONE',  ( -10.19494410001831497, 9.858401829237468661, 33.01259202755186095 ) ) ;
#5045=VERTEX_POINT ( 'NONE', #5149 ) ;
#5047=CARTESIAN_POINT ( 'NONE',  ( -6.095889600840176392, -10.32655419438761868, 28.09296952102860345 ) ) ;
#5049=FACE_OUTER_BOUND ( 'NONE', #3215, .T. ) ;
#5056=CARTESIAN_POINT ( 'NONE',  ( -9.900940235153615987, -0.8289898103093424897, 22.73823205004162418 ) ) ;
#5062=CARTESIAN_POINT ( 'NONE',  ( 0.000000000000000000, 0.000000000000000000, 38.00000000000000000 ) ) ;
#5065=CARTESIAN_POINT ( 'NONE',  ( 11.71455171164206988, -6.400535080091636964, 33.18278799730941842 ) ) ;
#5067=CARTESIAN_POINT ( 'NONE',  ( -10.50531938289192624, 7.869812776064899928, 30.57803900350706883 ) ) ;
#5070=CARTESIAN_POINT ( 'NONE',  ( -6.400384853991316625, 11.71459457793454817, 33.18278774224378225 ) ) ;
#5071=LINE ( 'NONE', #225, #4723 ) ;
#5080=CARTESIAN_POINT ( 'NONE',  ( -5.954811582427138816, -9.638809502600512502, 25.54535933516314472 ) ) ;
#5082=LINE ( 'NONE', #4575, #297 ) ;
#5088=CARTESIAN_POINT ( 'NONE',  ( 10.00265588554886165, -10.00265588554885099, 33.03935750738956756 ) ) ;
#5094=CARTESIAN_POINT ( 'NONE',  ( 11.79779776130986058, -1.839547822007355782, 30.71783115363462358 ) ) ;
#5095=CARTESIAN_POINT ( 'NONE',  ( -13.50805179034379044, 5.845970755595364388, 38.28811402100272687 ) ) ;
#5097=CARTESIAN_POINT ( 'NONE',  ( -2.742560498089726018, 11.69030472852370650, 30.70728637550628548 ) ) ;
#5102=CARTESIAN_POINT ( 'NONE',  ( -14.48620990986885637, 2.403201876585511432, 38.17751351274290528 ) ) ;
#5104=LINE ( 'NONE', #2726, #2476 ) ;
#5109=DIRECTION ( 'NONE',  ( 0.000000000000000000, 0.000000000000000000, 1.000000000000000000 ) ) ;
#5111=CARTESIAN_POINT ( 'NONE',  ( -15.67638808697554786, -1.082228759108213589, 38.00000000000000711 ) ) ;
#5118=SHAPE_REPRESENTATION_RELATIONSHIP ( 'NONE' , 'NONE' ,  #5596, #5819 ) ;
#5119=CARTESIAN_POINT ( 'NONE',  ( 13.50805179034378689, -5.845970755595367052, 38.28811402100272687 ) ) ;
#5121=CARTESIAN_POINT ( 'NONE',  ( -8.964415574088988592, 6.652784304366588408, 22.96342341013486887 ) ) ;
#5123=CARTESIAN_POINT ( 'NONE',  ( -1.902479615894477005, 12.74240908541723805, 33.26151609189631841 ) ) ;
#5130=LINE ( 'NONE', #2255, #4224 ) ;
#5131=CARTESIAN_POINT ( 'NONE',  ( -12.71058384521454521, 7.353037798771222100, 38.12486502407010391 ) ) ;
#5134=CARTESIAN_POINT ( 'NONE',  ( -8.321939193476740826, -8.970286671637149212, 22.89273732682886831 ) ) ;
#5135=AXIS2_PLACEMENT_3D ( 'NONE', #5200, #4286, #4792 ) ;
#5144=CARTESIAN_POINT ( 'NONE',  ( -9.999999999999998224, -9.166666666666657193, 23.00000000000000000 ) ) ;
#5146=FACE_OUTER_BOUND ( 'NONE', #5698, .T. ) ;
#5149=CARTESIAN_POINT ( 'NONE',  ( -8.999999999999998224, -8.999999999999998224, -167.0000000000000284 ) ) ;
#5151=CARTESIAN_POINT ( 'NONE',  ( -8.930195544527062879, 11.65680117706474661, 38.09189898655662887 ) ) ;
#5152=ADVANCED_FACE ( 'NONE', ( #5677, #4775 ), #18, .T. ) ;
#5153=CARTESIAN_POINT ( 'NONE',  ( 14.74111653287705614, 1.016991241531505441, 38.35393095385146012 ) ) ;
#5156=CARTESIAN_POINT ( 'NONE',  ( -1.776762854451772400, 10.85316926984840791, 28.17414535953233923 ) ) ;
#5158=CARTESIAN_POINT ( 'NONE',  ( -9.999999999999998224, 9.999999999999998224, 23.00000000000000000 ) ) ;
#5164=AXIS2_PLACEMENT_3D ( 'NONE', #5929, #1527, #4458 ) ;
#5166=CARTESIAN_POINT ( 'NONE',  ( -7.392961014695934807, -12.01622299351614487, 35.69843844696170976 ) ) ;
#5176=EDGE_CURVE ( 'NONE', #4467, #5045, #198, .T. ) ;
#5181=DIRECTION ( 'NONE',  ( 0.000000000000000000, 1.000000000000000000, 0.000000000000000000 ) ) ;
#5183=CARTESIAN_POINT ( 'NONE',  ( 12.81596724893641337, -2.042222512990850616E-14, 33.26667497053200151 ) ) ;
#5187=CARTESIAN_POINT ( 'NONE',  ( -4.666802875123988947, 12.24718835365691305, 33.22501703466258505 ) ) ;
#5193=CARTESIAN_POINT ( 'NONE',  ( -10.67327843797380815, -8.785602912694960409, 33.09221060678261495 ) ) ;
#5194=CARTESIAN_POINT ( 'NONE',  ( -12.46477214039063597, 7.762281575598230177, 38.11692635423788289 ) ) ;
#5200=CARTESIAN_POINT ( 'NONE',  ( 0.000000000000000000, 0.000000000000000000, 205.0000000000000568 ) ) ;
#5201=DIRECTION ( 'NONE',  ( -0.000000000000000000, -0.000000000000000000, -1.000000000000000000 ) ) ;
#5204=CARTESIAN_POINT ( 'NONE',  ( 8.539045536263008884, -9.793778397576030414, 27.99842134739335364 ) ) ;
#5215=B_SPLINE_CURVE_WITH_KNOTS ( 'NONE', 3,
 ( #1776, #2275, #2304, #3698, #2715, #4613, #5585, #4194, #5559, #365, #864, #2805, #4702, #453, #2744, #4079, #5994, #2777, #1707, #839, #5526, #5644, #5151, #4142, #3184, #1311 ),
 .UNSPECIFIED., .F., .F.,
 ( 4, 2, 2, 2, 2, 2, 2, 2, 2, 2, 2, 2, 4 ),
 ( 0.000000000000000000, 0.002857484983890443489, 0.004286227475835666101, 0.005714969967780886978, 0.008572454951671333936, 0.01000119744361655655, 0.01142993993556177743, 0.01428742491945222091, 0.01571616741139744353, 0.01714490990334266440, 0.02000239488723310963, 0.02143113737917832703, 0.02285987987112354444 ),
 .UNSPECIFIED. ) ;
#5216=B_SPLINE_CURVE_WITH_KNOTS ( 'NONE', 3,
 ( #115, #628, #717, #2506, #2057, #2534 ),
 .UNSPECIFIED., .F., .F.,
 ( 4, 2, 4 ),
 ( 2.991083242018516676E-05, 0.007589224902226409351, 0.01514853897203263453 ),
 .UNSPECIFIED. ) ;
#5218=CARTESIAN_POINT ( 'NONE',  ( 2.570253631893349766, 9.871311131128940985, 25.61911440830482789 ) ) ;
#5219=CARTESIAN_POINT ( 'NONE',  ( 9.999999999999998224, 8.333333333333316162, 23.00000000000000000 ) ) ;
#5224=FACE_OUTER_BOUND ( 'NONE', #4304, .T. ) ;
#5226=CARTESIAN_POINT ( 'NONE',  ( 9.981067540164714202, -9.981067540164714202, 22.73823205004162773 ) ) ;
#5228=VECTOR ( 'NONE', #5201, 1000.000000000000000 ) ;
#5229=CARTESIAN_POINT ( 'NONE',  ( -10.00265588554884744, 10.00265588554886165, 33.03935750738952493 ) ) ;
#5238=EDGE_LOOP ( 'NONE', ( #1891, #2792, #4479, #657 ) ) ;
#5239=FACE_OUTER_BOUND ( 'NONE', #488, .T. ) ;
#5240=CARTESIAN_POINT ( 'NONE',  ( 9.618700053625529378, -10.13908112636436520, 30.46372964425718521 ) ) ;
#5241=CARTESIAN_POINT ( 'NONE',  ( 4.273103006804781501, -9.778265433844634202, 25.59105575288734968 ) ) ;
#5253=CARTESIAN_POINT ( 'NONE',  ( 3.322922547535530846, 8.964120815521452457, 23.06129036953744915 ) ) ;
#5254=CARTESIAN_POINT ( 'NONE',  ( 5.273949241992681891, 14.79903580929012108, 38.00000000000000711 ) ) ;
#5255=CARTESIAN_POINT ( 'NONE',  ( -14.30354638250589794, -3.321916882804577753, 38.17191617598168563 ) ) ;
#5259=CARTESIAN_POINT ( 'NONE',  ( -8.975362584346067152, -9.157688896001735301, 22.85246612729342885 ) ) ;
#5261=EDGE_CURVE ( 'NONE', #3300, #4909, #1431, .T. ) ;
#5262=CARTESIAN_POINT ( 'NONE',  ( -9.144590365090035533, -9.969668718019493170, 22.73823205004162773 ) ) ;
#5269=ORIENTED_EDGE ( 'NONE', *, *, #248, .T. ) ;
#5272=CARTESIAN_POINT ( 'NONE',  ( 9.999999999999998224, 9.999999999999998224, 23.00000000000000000 ) ) ;
#5275=CARTESIAN_POINT ( 'NONE',  ( 9.994658916190591214, -8.983694681928700021, 22.80938439471026058 ) ) ;
#5283=FACE_OUTER_BOUND ( 'NONE', #3594, .T. ) ;
#5284=ORIENTED_EDGE ( 'NONE', *, *, #5261, .F. ) ;
#5285=CARTESIAN_POINT ( 'NONE',  ( 0.8304760625349936198, 8.965668681055126044, 23.09216300389308074 ) ) ;
#5286=CARTESIAN_POINT ( 'NONE',  ( 8.069545871843432749, 13.47611570251764768, 37.99999999999999289 ) ) ;
#5290=CARTESIAN_POINT ( 'NONE',  ( -13.11530391917000316, -6.736970939972939831, 38.26632377370044225 ) ) ;
#5291=CARTESIAN_POINT ( 'NONE',  ( -1.666666666666713814, -9.999999999999998224, 23.00000000000000000 ) ) ;
#5297=DIRECTION ( 'NONE',  ( 0.000000000000000000, 0.000000000000000000, 1.000000000000000000 ) ) ;
#5302=CARTESIAN_POINT ( 'NONE',  ( 6.736970939972923844, -13.11530391917000316, 38.26632377370044935 ) ) ;
#5310=CARTESIAN_POINT ( 'NONE',  ( 8.983694681928700021, -9.994658916190592990, 22.80938439471025703 ) ) ;
#5312=CARTESIAN_POINT ( 'NONE',  ( 1.016991241531516987, 14.74111653287705792, 38.35393095385146012 ) ) ;
#5313=CARTESIAN_POINT ( 'NONE',  ( 11.08488032081242203, 11.08488032081242203, 38.00000000000000000 ) ) ;
#5315=ORIENTED_EDGE ( 'NONE', *, *, #1680, .T. ) ;
#5317=CARTESIAN_POINT ( 'NONE',  ( -12.74242197681752309, 1.902388932222470963, 33.26151580524048512 ) ) ;
#5319=CARTESIAN_POINT ( 'NONE',  ( 0.8333333333332849646, -10.00000000000000000, 23.00000000000000355 ) ) ;
#5330=CARTESIAN_POINT ( 'NONE',  ( 0.000000000000000000, 0.000000000000000000, 38.00000000000000000 ) ) ;
#5331=CARTESIAN_POINT ( 'NONE',  ( 9.322893336083156512, -9.590870124851306855, 27.95908392747358917 ) ) ;
#5337=CARTESIAN_POINT ( 'NONE',  ( 11.04414289254854253, 9.677595944628125224, 38.07286884698773832 ) ) ;
#5343=CARTESIAN_POINT ( 'NONE',  ( 10.99573437649350005, -9.772747244158503932, 38.14042781937035187 ) ) ;
#5348=CARTESIAN_POINT ( 'NONE',  ( 0.9193131588476516347, 11.85339260696609287, 30.72304697887226510 ) ) ;
#5353=CARTESIAN_POINT ( 'NONE',  ( -12.81596724893641337, 0.9505942623812192460, 33.26667497053200151 ) ) ;
#5357=CARTESIAN_POINT ( 'NONE',  ( 8.964120776013636771, 3.322926169935025431, 23.06129021161080317 ) ) ;
#5361=CARTESIAN_POINT ( 'NONE',  ( -14.67638808697554964, 0.000000000000000000, 205.0000000000000568 ) ) ;
#5363=B_SPLINE_CURVE_WITH_KNOTS ( 'NONE', 3,
 ( #4068, #5985, #735, #1697, #5514, #1242 ),
 .UNSPECIFIED., .F., .F.,
 ( 4, 2, 4 ),
 ( 0.002357188415687244253, 0.01135824717474481077, 0.02035930593380237685 ),
 .UNSPECIFIED. ) ;
#5368=CARTESIAN_POINT ( 'NONE',  ( -3.322922547535532178, -8.964120815521452457, 23.06129036953745270 ) ) ;
#5371=DIRECTION ( 'NONE',  ( -0.07194996680737208994, 0.07194996680737265893, -0.9948097328398211037 ) ) ;
#5373=VECTOR ( 'NONE', #1433, 1000.000000000000000 ) ;
#5379=ORIENTED_EDGE ( 'NONE', *, *, #1051, .F. ) ;
#5381=CARTESIAN_POINT ( 'NONE',  ( 9.939337621248920840, -6.642184745761470666, 22.73823205004162418 ) ) ;
#5386=CARTESIAN_POINT ( 'NONE',  ( -12.74411457810409409, -5.685785403169723473, 35.74643938915853880 ) ) ;
#5388=CARTESIAN_POINT ( 'NONE',  ( 4.260267006495011444, -15.12434353048566571, 38.00000000000000711 ) ) ;
#5394=CARTESIAN_POINT ( 'NONE',  ( -4.532931003857846086, -11.42336634021359387, 30.68084270896568810 ) ) ;
#5395=VERTEX_POINT ( 'NONE', #3133 ) ;
#5396=DIRECTION ( 'NONE',  ( 1.000000000000000000, 0.000000000000000000, 0.000000000000000000 ) ) ;
#5402=CARTESIAN_POINT ( 'NONE',  ( -9.981067540164714202, -9.981067540164714202, 22.73823205004162418 ) ) ;
#5404=CARTESIAN_POINT ( 'NONE',  ( 10.38144361273100635, 10.38144361273100458, 38.10175261887127363 ) ) ;
#5405=CARTESIAN_POINT ( 'NONE',  ( 9.910574073276151807, 3.317157231508560677, 22.73823205004162418 ) ) ;
#5411=CARTESIAN_POINT ( 'NONE',  ( -12.24718835365690417, -4.666802875123986283, 33.22501703466257794 ) ) ;
#5415=CARTESIAN_POINT ( 'NONE',  ( 9.833810162157899271, 3.423816715609354855, 25.60794618818621160 ) ) ;
#5420=CARTESIAN_POINT ( 'NONE',  ( 1.968147360634805443, -13.68731696136523546, 35.80501325620552677 ) ) ;
#5423=VECTOR ( 'NONE', #1922, 1000.000000000000000 ) ;
#5430=CARTESIAN_POINT ( 'NONE',  ( 0.000000000000000000, 0.000000000000000000, 205.0000000000000568 ) ) ;
#5435=CARTESIAN_POINT ( 'NONE',  ( 9.902916272933978803, 1.657983872361815658, 22.73823205004162418 ) ) ;
#5437=CIRCLE ( 'NONE', #4120, 15.67638808697555142 ) ;
#5443=CARTESIAN_POINT ( 'NONE',  ( -8.965668681055127820, 0.8304760625349917325, 23.09216300389307719 ) ) ;
#5446=CARTESIAN_POINT ( 'NONE',  ( -9.245260337044125976, 9.269614772507654976, 25.40693856330804223 ) ) ;
#5450=CARTESIAN_POINT ( 'NONE',  ( 9.638809746143360613, 5.954763795926134584, 25.54536317066255791 ) ) ;
#5454=CARTESIAN_POINT ( 'NONE',  ( -6.000509662810409317, 9.000000000000001776, 23.13502399099478524 ) ) ;
#5458=EDGE_CURVE ( 'NONE', #2297, #4386, #2614, .T. ) ;
#5459=CARTESIAN_POINT ( 'NONE',  ( -2.654236408786764034, -10.78034266696900367, 28.16346921039841789 ) ) ;
#5460=VERTEX_POINT ( 'NONE', #4714 ) ;
#5473=CARTESIAN_POINT ( 'NONE',  ( 7.077172123266715964, 10.77715421822219355, 30.61076540981938976 ) ) ;
#5474=CARTESIAN_POINT ( 'NONE',  ( 15.67638808697554431, 1.082228759108213367, 38.00000000000000000 ) ) ;
#5475=DIRECTION ( 'NONE',  ( 1.000000000000000000, 0.000000000000000000, 0.000000000000000000 ) ) ;
#5478=CARTESIAN_POINT ( 'NONE',  ( -9.462636878983097688, 7.610208295502505216, 25.48187184588751464 ) ) ;
#5480=CARTESIAN_POINT ( 'NONE',  ( -10.38144361273100458, 10.38144361273100635, 38.10175261887127363 ) ) ;
#5482=CARTESIAN_POINT ( 'NONE',  ( 12.64046943599297101, 7.570233152424905576, 38.23931941266579315 ) ) ;
#5485=CARTESIAN_POINT ( 'NONE',  ( -8.309552794738946702, 9.958856949317492990, 22.73823205004162418 ) ) ;
#5487=CARTESIAN_POINT ( 'NONE',  ( -9.999999999999998224, 9.999999999999998224, 23.00000000000000000 ) ) ;
#5488=CARTESIAN_POINT ( 'NONE',  ( -0.8880320553140829132, -10.89081796499577237, 28.17941898721253935 ) ) ;
#5499=CARTESIAN_POINT ( 'NONE',  ( 10.27356722921338772, 10.12138240269938905, 35.55812462721154787 ) ) ;
#5505=CARTESIAN_POINT ( 'NONE',  ( -11.12726264164139600, 8.926511697459378780, 35.63515070857870626 ) ) ;
#5511=CARTESIAN_POINT ( 'NONE',  ( -8.333333333333316162, 9.999999999999998224, 23.00000000000000000 ) ) ;
#5512=CARTESIAN_POINT ( 'NONE',  ( -5.113933401365549081, -9.708537589994012507, 25.56820946177495912 ) ) ;
#5514=CARTESIAN_POINT ( 'NONE',  ( -8.999999999999992895, -6.000509662810403100, 23.13502399099456142 ) ) ;
#5515=ORIENTED_EDGE ( 'NONE', *, *, #3039, .T. ) ;
#5517=FACE_OUTER_BOUND ( 'NONE', #4767, .T. ) ;
#5519=CARTESIAN_POINT ( 'NONE',  ( -9.930636381741159369, -5.809855716632609024, 22.73823205004162418 ) ) ;
#5526=CARTESIAN_POINT ( 'NONE',  ( -7.333173243373228622, 12.74975250248360936, 38.12600698484704509 ) ) ;
#5530=ORIENTED_EDGE ( 'NONE', *, *, #2250, .T. ) ;
#5531=CARTESIAN_POINT ( 'NONE',  ( 13.11522978513662707, -6.737147714782516950, 38.26633100282688105 ) ) ;
#5534=CARTESIAN_POINT ( 'NONE',  ( -9.933255351449997050, 9.419333092093008730, 30.50691708577705796 ) ) ;
#5536=CARTESIAN_POINT ( 'NONE',  ( -9.322893336083152960, 9.590870124851306855, 27.95908392747358917 ) ) ;
#5538=B_SPLINE_SURFACE_WITH_KNOTS ( 'NONE', 3, 3, ( 
 ( #4310, #613, #1388, #2492, #3381, #6126, #1848 ),
 ( #514, #2391, #3745, #2820, #1419, #4281, #4720 ),
 ( #5692, #3318, #1154, #754, #1212, #3075, #3102 ),
 ( #5821, #3972, #5914, #4950, #2040, #3999, #2009 ),
 ( #5482, #1628, #1545, #3477, #3534, #3564, #4981 ),
 ( #2072, #3010, #1604, #5009, #4409, #5450, #1182 ),
 ( #728, #2610, #4500, #2129, #254, #702, #4027 ),
 ( #1130, #4473, #5947, #4894, #3940, #5858, #3501 ),
 ( #4379, #3904, #642, #3447, #2582, #5415, #5357 ),
 ( #1105, #196, #3041, #2984, #226, #2521, #156 ),
 ( #1578, #4919, #669, #2552, #4441, #6082, #2779 ),
 ( #5153, #5562, #2716, #427, #4676, #3644, #4646 ),
 ( #3185, #2306, #5183, #2749, #1286, #1312, #4614 ),
 ( #1746, #814, #369, #4143, #2277, #4170, #3157 ),
 ( #399, #5997, #1711, #5094, #840, #5650, #341 ),
 ( #3612, #4195, #5611, #6112, #1342, #2247, #6057 ),
 ( #3213, #1375, #1778, #2216, #3673, #1803, #314 ),
 ( #3279, #865, #3699, #4107, #3248, #900, #5587 ),
 ( #5119, #1831, #3732, #925, #4557, #2192, #4083 ),
 ( #5531, #1259, #5065, #2689, #4588, #6026, #2475 ),
 ( #2839, #3793, #1502, #1407, #3306, #3827, #3398 ),
 ( #4330, #1964, #3864, #595, #1053, #3370, #2436 ),
 ( #3892, #2379, #2931, #4779, #4744, #1870, #5808 ),
 ( #5343, #5746, #4842, #532, #497, #2410, #4366 ),
 ( #116, #4298, #47, #5240, #1926, #5781, #5310 ) ),
 .UNSPECIFIED., .F., .F., .F.,
 ( 4, 3, 3, 3, 3, 3, 3, 3, 4 ),
 ( 4, 3, 4 ),
 ( 0.000000000000000000, 0.1250000000000000000, 0.2500000000000000000, 0.3750000000000000000, 0.5000000000000000000, 0.6250000000000000000, 0.7500000000000000000, 0.8750000000000000000, 1.000000000000000000 ),
 ( 0.000000000000000000, 0.5087255983319458608, 1.017451196663891722 ),
 .UNSPECIFIED. ) ;
#5545=CARTESIAN_POINT ( 'NONE',  ( -5.390571672161876826, -11.22195964661421819, 30.65936073406735218 ) ) ;
#5553=CARTESIAN_POINT ( 'NONE',  ( -9.902916272933978803, -1.657983872361813660, 22.73823205004162418 ) ) ;
#5559=CARTESIAN_POINT ( 'NONE',  ( 3.819063922342337047, 14.20304409106728727, 38.16887386538297733 ) ) ;
#5561=ADVANCED_FACE ( 'NONE', ( #1 ), #4586, .T. ) ;
#5562=CARTESIAN_POINT ( 'NONE',  ( 13.77854189090673387, 0.9833031778629049979, 35.81030296219172726 ) ) ;
#5563=CARTESIAN_POINT ( 'NONE',  ( -9.269614772507654976, 9.245260337044141963, 25.40693856330804223 ) ) ;
#5565=CARTESIAN_POINT ( 'NONE',  ( -3.322926169935024987, 8.964120776013636771, 23.06129021161080317 ) ) ;
#5573=CARTESIAN_POINT ( 'NONE',  ( -8.662453428863081228, -10.23348454756166070, 30.54531259719474079 ) ) ;
#5580=CARTESIAN_POINT ( 'NONE',  ( -15.12434353048566571, 4.260267006495016773, 38.00000000000000711 ) ) ;
#5585=CARTESIAN_POINT ( 'NONE',  ( 6.075059976386698146, 13.36876581604897574, 38.14410695834214948 ) ) ;
#5587=CARTESIAN_POINT ( 'NONE',  ( 8.963431154120575783, -4.154433491267528034, 23.04275521548131067 ) ) ;
#5588=CARTESIAN_POINT ( 'NONE',  ( -12.64059746256322647, 7.570044180282075708, 38.23931193745812607 ) ) ;
#5590=CARTESIAN_POINT ( 'NONE',  ( -8.785602912694963962, 10.67327843797381171, 33.09221060678261495 ) ) ;
#5596=SHAPE_REPRESENTATION ( 'tube', ( #73 ), #684 ) ;
#5597=CARTESIAN_POINT ( 'NONE',  ( -7.732441893382042686, -9.977717576970372093, 28.03187055541260264 ) ) ;
#5605=CARTESIAN_POINT ( 'NONE',  ( -9.958856949317492990, 8.309552794738976900, 22.73823205004162418 ) ) ;
#5611=CARTESIAN_POINT ( 'NONE',  ( 12.60026679007841643, -2.830884587392778595, 33.25110354061416729 ) ) ;
#5613=CARTESIAN_POINT ( 'NONE',  ( -10.12138240269938727, 10.27356722921339127, 35.55812462721154787 ) ) ;
#5614=ORIENTED_EDGE ( 'NONE', *, *, #3645, .T. ) ;
#5627=CARTESIAN_POINT ( 'NONE',  ( -9.994658916190592990, -8.983694681928700021, 22.80938439471026058 ) ) ;
#5631=ORIENTED_EDGE ( 'NONE', *, *, #1398, .F. ) ;
#5637=EDGE_CURVE ( 'NONE', #5798, #1401, #5071, .T. ) ;
#5640=CARTESIAN_POINT ( 'NONE',  ( 10.37777353962609972, -10.37777353962564852, 38.05103295300747845 ) ) ;
#5644=CARTESIAN_POINT ( 'NONE',  ( -8.540366387015959404, 11.94538915683136793, 38.10041598230911575 ) ) ;
#5645=DIRECTION ( 'NONE',  ( 1.000000000000000000, 0.000000000000000000, 0.000000000000000000 ) ) ;
#5650=CARTESIAN_POINT ( 'NONE',  ( 9.908812303639313868, -1.716658579843636678, 25.63028407385522911 ) ) ;
#5653=ORIENTED_EDGE ( 'NONE', *, *, #5637, .T. ) ;
#5660=CARTESIAN_POINT ( 'NONE',  ( -9.269614772507654976, -9.245260337044127752, 25.40693856330804223 ) ) ;
#5677=FACE_OUTER_BOUND ( 'NONE', #323, .T. ) ;
#5679=CARTESIAN_POINT ( 'NONE',  ( 10.00265588554886165, 10.00265588554885632, 33.03935750738954624 ) ) ;
#5683=CARTESIAN_POINT ( 'NONE',  ( -6.736970939972922956, 13.11530391916999960, 38.26632377370044935 ) ) ;
#5690=CARTESIAN_POINT ( 'NONE',  ( -13.37091851167933854, 6.070355506014839975, 38.14417062278695170 ) ) ;
#5692=CARTESIAN_POINT ( 'NONE',  ( 11.58129469348872931, 9.086808451283779675, 38.17632780249462598 ) ) ;
#5693=CARTESIAN_POINT ( 'NONE',  ( -0.9766276285323429729, -14.65181115585165372, 38.18271774125523876 ) ) ;
#5694=ORIENTED_EDGE ( 'NONE', *, *, #3998, .T. ) ;
#5698=EDGE_LOOP ( 'NONE', ( #298, #2941, #3059, #2035 ) ) ;
#5699=CARTESIAN_POINT ( 'NONE',  ( 13.92731518891505438, -4.729006349282931509, 38.16144984630090420 ) ) ;
#5700=CARTESIAN_POINT ( 'NONE',  ( 6.095798759547082390, -10.32656711695237739, 28.09297316833069402 ) ) ;
#5706=CARTESIAN_POINT ( 'NONE',  ( 8.999999999988068211, 9.000000000000005329, 23.06137295785747554 ) ) ;
#5711=CARTESIAN_POINT ( 'NONE',  ( 5.685785403169734131, 12.74411457810409409, 35.74643938915853880 ) ) ;
#5712=CARTESIAN_POINT ( 'NONE',  ( 5.809855716632679190, 9.930636381741159369, 22.73823205004162418 ) ) ;
#5713=CARTESIAN_POINT ( 'NONE',  ( -13.74495680931371666, -5.167291852658159712, 38.15579506865710613 ) ) ;
#5714=ORIENTED_EDGE ( 'NONE', *, *, #3493, .F. ) ;
#5718=CARTESIAN_POINT ( 'NONE',  ( -9.977717576970366764, -7.732441893382013376, 28.03187055541259554 ) ) ;
#5725=CARTESIAN_POINT ( 'NONE',  ( -1.937269431830245248, -14.55597330376941123, 38.18000980160655899 ) ) ;
#5730=DIRECTION ( 'NONE',  ( 1.000000000000000000, 0.000000000000000000, 0.000000000000000000 ) ) ;
#5735=CARTESIAN_POINT ( 'NONE',  ( 9.632247231687289357, -10.63625351335941538, 35.59852902770369099 ) ) ;
#5740=LINE ( 'NONE', #526, #3959 ) ;
#5741=CARTESIAN_POINT ( 'NONE',  ( -9.999999999999998224, 9.999999999999998224, -167.0000000000000284 ) ) ;
#5746=CARTESIAN_POINT ( 'NONE',  ( 10.63625351335941538, -9.632247231687294686, 35.59852902770369809 ) ) ;
#5748=CARTESIAN_POINT ( 'NONE',  ( 2.780685750889414288E-14, 9.928243323025453648, 25.63579099555277807 ) ) ;
#5749=CARTESIAN_POINT ( 'NONE',  ( 9.144590365090033757, 9.969668718019493170, 22.73823205004162418 ) ) ;
#5752=ORIENTED_EDGE ( 'NONE', *, *, #2593, .T. ) ;
#5755=CARTESIAN_POINT ( 'NONE',  ( -10.27564057804868725, -9.515772848102848513, 33.05475024408053031 ) ) ;
#5758=CARTESIAN_POINT ( 'NONE',  ( 5.833333333333301063, -9.999999999999998224, 23.00000000000000000 ) ) ;
#5763=CARTESIAN_POINT ( 'NONE',  ( 8.540366387015776439, -11.94538915683149582, 38.10041598230914417 ) ) ;
#5764=CIRCLE ( 'NONE', #1001, 15.67638808697555142 ) ;
#5771=CARTESIAN_POINT ( 'NONE',  ( 7.228764404800513965, -11.39256393965315795, 33.15620429642044797 ) ) ;
#5772=APPLICATION_CONTEXT ( 'automotive_design' ) ;
#5774=CARTESIAN_POINT ( 'NONE',  ( -9.166555234036119160, 10.04707028972858929, 25.36260747786040071 ) ) ;
#5777=CARTESIAN_POINT ( 'NONE',  ( 0.000000000000000000, 0.000000000000000000, -167.0000000000000284 ) ) ;
#5781=CARTESIAN_POINT ( 'NONE',  ( 9.166555234036119160, -10.04707028972858929, 25.36260747786040071 ) ) ;
#5783=CARTESIAN_POINT ( 'NONE',  ( 3.645573174172184849, 11.58281169573756131, 30.69674159737795449 ) ) ;
#5784=CARTESIAN_POINT ( 'NONE',  ( 8.333333333333348136, 9.999999999999998224, 23.00000000000000000 ) ) ;
#5788=CARTESIAN_POINT ( 'NONE',  ( -11.58129469348872398, -9.086808451283777899, 38.17632780249461888 ) ) ;
#5792=CARTESIAN_POINT ( 'NONE',  ( -3.000437278975514044, -9.000000000000001776, 23.18288419282211876 ) ) ;
#5793=DIRECTION ( 'NONE',  ( 1.000000000000000000, 0.000000000000000000, 0.000000000000000000 ) ) ;
#5796=CARTESIAN_POINT ( 'NONE',  ( 9.999999999999998224, -9.999999999999998224, 23.00000000000000000 ) ) ;
#5798=VERTEX_POINT ( 'NONE', #3285 ) ;
#5800=DIRECTION ( 'NONE',  ( 0.000000000000000000, 0.000000000000000000, 1.000000000000000000 ) ) ;
#5802=CARTESIAN_POINT ( 'NONE',  ( 7.487361748921619764, -8.967351122863068014, 22.92808036848186859 ) ) ;
#5807=CARTESIAN_POINT ( 'NONE',  ( -9.999999999999996447, -9.999999999999996447, 22.99999999999995737 ) ) ;
#5808=CARTESIAN_POINT ( 'NONE',  ( 8.970286671637149212, -8.321939193476740826, 22.89273732682886475 ) ) ;
#5810=CARTESIAN_POINT ( 'NONE',  ( -0.8304760625348921455, 8.965668681055129596, 23.09216300389309140 ) ) ;
#5812=CARTESIAN_POINT ( 'NONE',  ( 9.999999999999998224, 9.999999999999998224, 23.00000000000000000 ) ) ;
#5813=VERTEX_POINT ( 'NONE', #5158 ) ;
#5815=CARTESIAN_POINT ( 'NONE',  ( -9.928243323025453648, 0.8581648076837686823, 25.63579099555280294 ) ) ;
#5818=CARTESIAN_POINT ( 'NONE',  ( 3.333333333333289961, -9.999999999999998224, 23.00000000000000000 ) ) ;
#5819=ADVANCED_BREP_SHAPE_REPRESENTATION ( '', ( #4119, #73 ), #684 ) ;
#5821=CARTESIAN_POINT ( 'NONE',  ( 12.11088206474084927, 8.328520801854342182, 38.20782360758020957 ) ) ;
#5822=CARTESIAN_POINT ( 'NONE',  ( 3.785572473853858089, -14.18798205797851075, 38.16905032409691501 ) ) ;
#5832=CARTESIAN_POINT ( 'NONE',  ( 10.19494410001831142, -9.858401829237472214, 33.01259202755186095 ) ) ;
#5848=CARTESIAN_POINT ( 'NONE',  ( 15.56315586465742840, -2.164213882025735280, 38.00000000000002132 ) ) ;
#5853=CARTESIAN_POINT ( 'NONE',  ( -14.74111653287705792, -1.016991241531516765, 38.35393095385146012 ) ) ;
#5855=CARTESIAN_POINT ( 'NONE',  ( -4.166666666666706931, -9.999999999999998224, 23.00000000000000000 ) ) ;
#5858=CARTESIAN_POINT ( 'NONE',  ( 9.778265433844637755, 4.273103006804793935, 25.59105575288735324 ) ) ;
#5859=AXIS2_PLACEMENT_3D ( 'NONE', #801, #2294, #4071 ) ;
#5866=CARTESIAN_POINT ( 'NONE',  ( -4.666652649023723676, -12.24723121994938957, 33.22501677959694177 ) ) ;
#5869=CARTESIAN_POINT ( 'NONE',  ( -9.999999999999998224, -9.999999999999998224, 23.00000000000000000 ) ) ;
#5871=CARTESIAN_POINT ( 'NONE',  ( 14.67638808697651953, 0.9595328539160939973, 38.18288438803428875 ) ) ;
#5875=FACE_OUTER_BOUND ( 'NONE', #4376, .T. ) ;
#5878=CARTESIAN_POINT ( 'NONE',  ( 8.328520801854336852, 12.11088206474084927, 38.20782360758020246 ) ) ;
#5884=CARTESIAN_POINT ( 'NONE',  ( -8.965240827029074211, -1.660911000355771883, 23.08598180255751942 ) ) ;
#5886=CARTESIAN_POINT ( 'NONE',  ( -8.069545871843436302, -13.47611570251764768, 37.99999999999999289 ) ) ;
#5892=CARTESIAN_POINT ( 'NONE',  ( 0.8304760625348978076, -8.965668681055127820, 23.09216300389306653 ) ) ;
#5895=EDGE_LOOP ( 'NONE', ( #3077, #3449, #2320, #3066 ) ) ;
#5896=CARTESIAN_POINT ( 'NONE',  ( 11.65565333135118209, 8.931668428567823170, 38.09186409098168014 ) ) ;
#5903=CARTESIAN_POINT ( 'NONE',  ( -9.999999999999998224, 9.999999999999998224, -167.0000000000000284 ) ) ;
#5904=CARTESIAN_POINT ( 'NONE',  ( 9.999999999999998224, 3.333333333333289961, 23.00000000000000000 ) ) ;
#5909=CARTESIAN_POINT ( 'NONE',  ( -8.965668681055127820, 4.802124745462707424E-14, 23.09216300389307719 ) ) ;
#5914=CARTESIAN_POINT ( 'NONE',  ( 11.03292118881348394, 8.007183658747743848, 33.12420745160152791 ) ) ;
#5917=CARTESIAN_POINT ( 'NONE',  ( 3.000437278975559785, 9.000000000000003553, 23.18288419282210810 ) ) ;
#5920=CARTESIAN_POINT ( 'NONE',  ( -3.423848683943053750, -9.833809958618578762, 25.60794474275443022 ) ) ;
#5929=CARTESIAN_POINT ( 'NONE',  ( 0.000000000000000000, 0.000000000000000000, 38.00000000000000000 ) ) ;
#5932=VERTEX_POINT ( 'NONE', #5812 ) ;
#5936=CARTESIAN_POINT ( 'NONE',  ( 9.900940235153617763, 0.8289898103093435999, 22.73823205004162773 ) ) ;
#5941=DIRECTION ( 'NONE',  ( 0.000000000000000000, 0.000000000000000000, -1.000000000000000000 ) ) ;
#5942=CARTESIAN_POINT ( 'NONE',  ( -10.78034266696899657, -2.654236408786700085, 28.16346921039841078 ) ) ;
#5944=EDGE_CURVE ( 'NONE', #4386, #251, #4854, .T. ) ;
#5947=CARTESIAN_POINT ( 'NONE',  ( 12.24718835365690772, 4.666802875123989836, 33.22501703466258505 ) ) ;
#5951=ORIENTED_EDGE ( 'NONE', *, *, #5944, .F. ) ;
#5953=CARTESIAN_POINT ( 'NONE',  ( -0.8304760625349921765, -8.965668681055127820, 23.09216300389308074 ) ) ;
#5956=DIRECTION ( 'NONE',  ( -1.000000000000000000, 0.000000000000000000, 0.000000000000000000 ) ) ;
#5962=DIRECTION ( 'NONE',  ( -0.000000000000000000, -0.000000000000000000, -1.000000000000000000 ) ) ;
#5966=CARTESIAN_POINT ( 'NONE',  ( 9.157688896001753065, 8.975362584346067152, 22.85246612729342885 ) ) ;
#5972=CARTESIAN_POINT ( 'NONE',  ( -12.41448144607148230, 6.563799387313612677, 35.72511331161845050 ) ) ;
#5975=CARTESIAN_POINT ( 'NONE',  ( -9.994658916190591214, 8.983694681928700021, 22.80938439471025703 ) ) ;
#5981=CARTESIAN_POINT ( 'NONE',  ( -8.069545871843429197, 13.47611570251764590, 37.99999999999999289 ) ) ;
#5983=CARTESIAN_POINT ( 'NONE',  ( 1.660911000355770106, -8.965240827029075987, 23.08598180255752297 ) ) ;
#5985=CARTESIAN_POINT ( 'NONE',  ( -8.999999999999996447, 6.000548030722253401, 23.13502304888919170 ) ) ;
#5991=CARTESIAN_POINT ( 'NONE',  ( -9.999999999999998224, 4.166666666666706931, 23.00000000000000000 ) ) ;
#5993=DIRECTION ( 'NONE',  ( -1.000000000000000000, 0.000000000000000000, 0.000000000000000000 ) ) ;
#5994=CARTESIAN_POINT ( 'NONE',  ( -3.785572473853681785, 14.18798205797855694, 38.16905032409690790 ) ) ;
#5997=CARTESIAN_POINT ( 'NONE',  ( 13.68733454931619775, -1.968046268140574151, 35.80501179064256689 ) ) ;
#5998=CARTESIAN_POINT ( 'NONE',  ( -10.63625351335941893, 9.632247231687291134, 35.59852902770369099 ) ) ;
#6000=CARTESIAN_POINT ( 'NONE',  ( -9.419333092092999848, 9.933255351449997050, 30.50691708577705796 ) ) ;
#6005=FACE_OUTER_BOUND ( 'NONE', #6061, .T. ) ;
#6006=CARTESIAN_POINT ( 'NONE',  ( -8.785766938566927919, -10.67320828294309898, 33.09220912812762094 ) ) ;
#6013=DIRECTION ( 'NONE',  ( 1.000000000000000000, 0.000000000000000000, 0.000000000000000000 ) ) ;
#6016=CARTESIAN_POINT ( 'NONE',  ( -9.910574073276151807, 3.317157231508650828, 22.73823205004162418 ) ) ;
#6019=ORIENTED_EDGE ( 'NONE', *, *, #3795, .T. ) ;
#6022=DIRECTION ( 'NONE',  ( 0.000000000000000000, 0.000000000000000000, 1.000000000000000000 ) ) ;
#6026=CARTESIAN_POINT ( 'NONE',  ( 9.638809502600501844, -5.954811582427137040, 25.54535933516314117 ) ) ;
#6028=CARTESIAN_POINT ( 'NONE',  ( -9.638809502600501844, 5.954811582427136152, 25.54535933516314472 ) ) ;
#6030=ORIENTED_EDGE ( 'NONE', *, *, #2746, .F. ) ;
#6031=ADVANCED_FACE ( 'NONE', ( #3610 ), #1205, .T. ) ;
#6032=CARTESIAN_POINT ( 'NONE',  ( -4.399300199984973681, 10.59948853791303947, 28.13666499103235097 ) ) ;
#6037=AXIS2_PLACEMENT_3D ( 'NONE', #3597, #205, #5956 ) ;
#6043=ORIENTED_EDGE ( 'NONE', *, *, #6065, .F. ) ;
#6047=VECTOR ( 'NONE', #4765, 999.9999999999998863 ) ;
#6049=CARTESIAN_POINT ( 'NONE',  ( -9.999999999999998224, -8.333333333333314386, 23.00000000000000000 ) ) ;
#6050=CARTESIAN_POINT ( 'NONE',  ( 9.000000000000005329, -8.999999999988066435, 23.06137295785747554 ) ) ;
#6051=VECTOR ( 'NONE', #5371, 999.9999999999998863 ) ;
#6054=PLANE ( 'NONE',  #2224 ) ;
#6057=CARTESIAN_POINT ( 'NONE',  ( 8.964680801521355491, -2.491918585145489029, 23.07363600708416129 ) ) ;
#6059=CARTESIAN_POINT ( 'NONE',  ( -11.22195964661421819, 5.390571672161876826, 30.65936073406735574 ) ) ;
#6061=EDGE_LOOP ( 'NONE', ( #1148, #4882, #1127, #260 ) ) ;
#6062=CARTESIAN_POINT ( 'NONE',  ( -5.819383256046894992, 8.963566061094550008, 22.99383858586042351 ) ) ;
#6065=EDGE_CURVE ( 'NONE', #2500, #6095, #5437, .T. ) ;
#6068=CARTESIAN_POINT ( 'NONE',  ( -10.13908112636436343, -9.618700053625529378, 30.46372964425718521 ) ) ;
#6075=CARTESIAN_POINT ( 'NONE',  ( -12.35760627049922178, 9.696021465980074083, 38.00000000000000000 ) ) ;
#6076=LINE ( 'NONE', #3639, #3259 ) ;
#6082=CARTESIAN_POINT ( 'NONE',  ( 9.908812100099982700, 1.716690548177159270, 25.63028262842344773 ) ) ;
#6083=CARTESIAN_POINT ( 'NONE',  ( -14.42236408824967775, 3.019346778933466258, 38.33740271606986738 ) ) ;
#6085=CARTESIAN_POINT ( 'NONE',  ( -6.563632016262921809, 12.41454131244163861, 35.72510948639917672 ) ) ;
#6090=CYLINDRICAL_SURFACE ( 'NONE', #2039, 15.67638808697555142 ) ;
#6093=EDGE_CURVE ( 'NONE', #936, #2868, #2042, .T. ) ;
#6094=CARTESIAN_POINT ( 'NONE',  ( -10.27356722921338950, -10.12138240269938727, 35.55812462721154787 ) ) ;
#6095=VERTEX_POINT ( 'NONE', #746 ) ;
#6103=ORIENTED_EDGE ( 'NONE', *, *, #6065, .T. ) ;
#6104=CARTESIAN_POINT ( 'NONE',  ( -9.969668718019493170, 9.144590365090033757, 22.73823205004162418 ) ) ;
#6107=CARTESIAN_POINT ( 'NONE',  ( -9.999999999999998224, -9.999999999999998224, -167.0000000000000284 ) ) ;
#6112=CARTESIAN_POINT ( 'NONE',  ( 11.69030472852371005, -2.742560498089769982, 30.70728637550628903 ) ) ;
#6115=CARTESIAN_POINT ( 'NONE',  ( -3.759289558891020455, 12.45812449473958949, 33.24069098933200195 ) ) ;
#6126=CARTESIAN_POINT ( 'NONE',  ( 9.166555234036119160, 10.04707028972859106, 25.36260747786040071 ) ) ;
#6128=CARTESIAN_POINT ( 'NONE',  ( -11.08488032081242025, 11.08488032081242203, 38.00000000000000000 ) ) ;
#6140=CARTESIAN_POINT ( 'NONE',  ( -11.03292118881348216, -8.007183658747740296, 33.12420745160152080 ) ) ;
#6171=COLOUR_RGB('Sky Blue',0.24,0.69,0.87);
#6172=FILL_AREA_STYLE_COLOUR('',#6171);
#6173=FILL_AREA_STYLE('',(#6172));
#6174=SURFACE_STYLE_FILL_AREA(#6173);
#6175=SURFACE_SIDE_STYLE('',(#6174));
#6176=SURFACE_STYLE_USAGE(.BOTH.,#6175);
#6177=PRESENTATION_STYLE_ASSIGNMENT((#6176));
ENDSEC;
END-ISO-10303-21;
